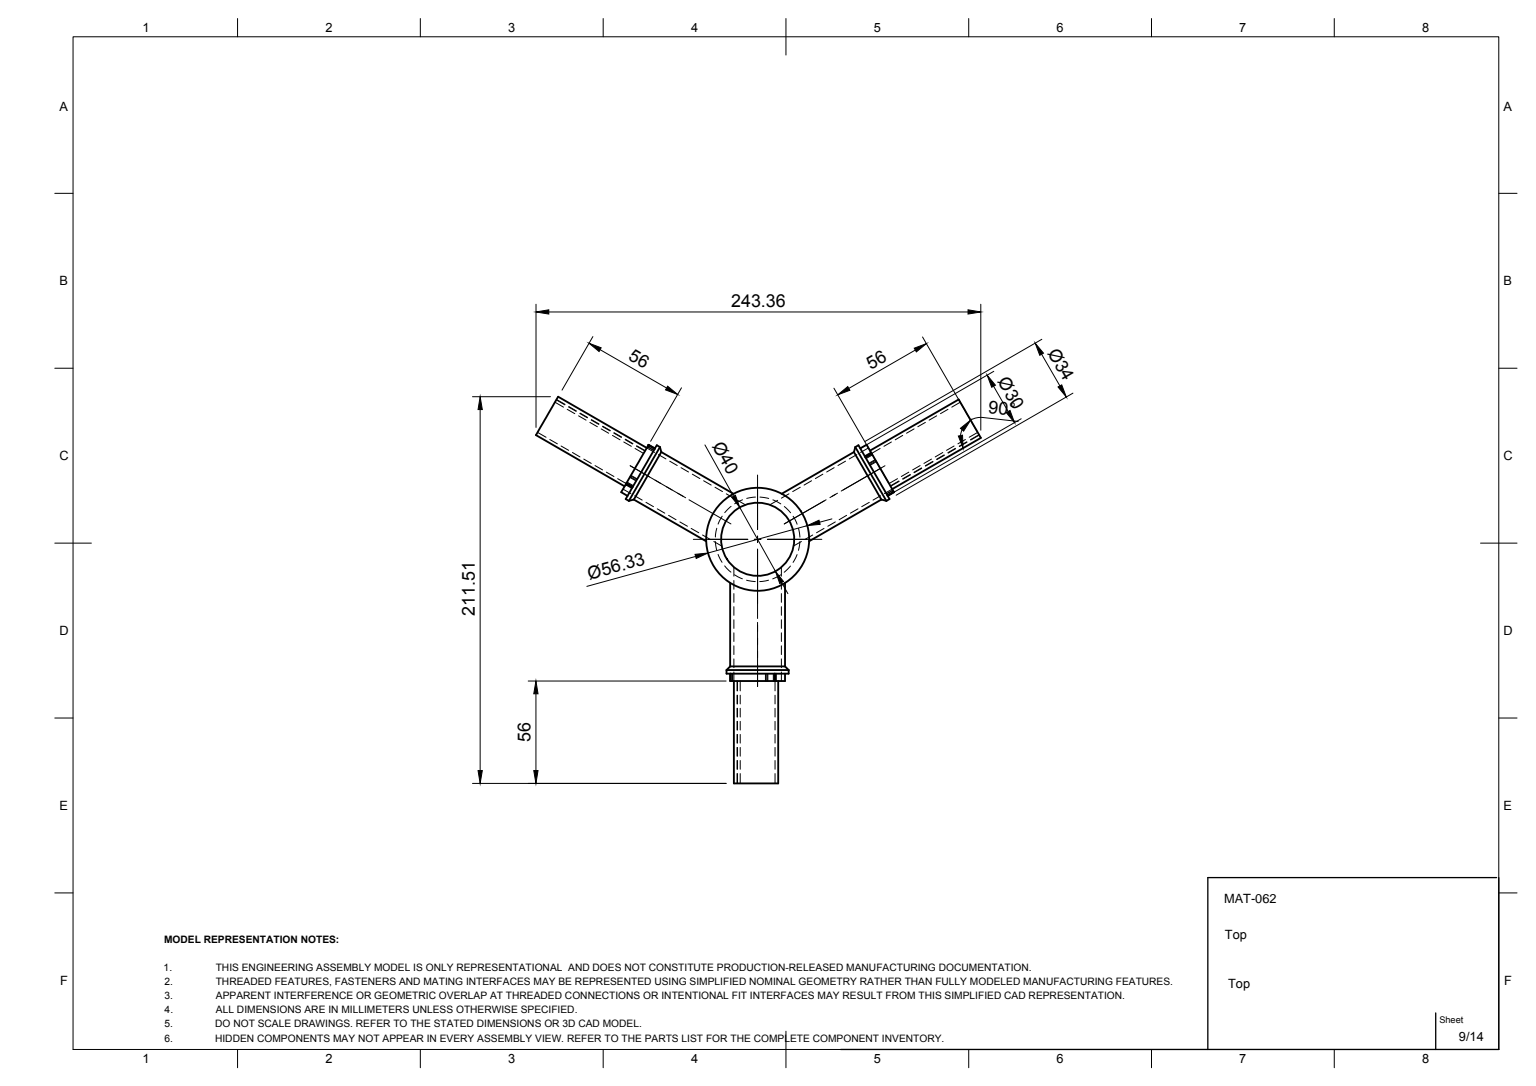
ISO-10303-21;
HEADER;
/* Generated by software containing ST-Developer
 * from STEP Tools, Inc. (www.steptools.com) 
 */

FILE_DESCRIPTION(
/* description */ (''),
/* implementation_level */ '2;1');

FILE_NAME(
/* name */ 'Top.step',
/* time_stamp */ '2026-10-24T10:18:25-07:00',
/* author */ (''),
/* organization */ (''),
/* preprocessor_version */ 'ST-DEVELOPER v20.2',
/* originating_system */ 'Autodesk Translation Framework v15.15.0.0',
/* authorisation */ '');

FILE_SCHEMA (('AUTOMOTIVE_DESIGN { 1 0 10303 214 3 1 1 }'));
ENDSEC;

DATA;
#10=MECHANICAL_DESIGN_GEOMETRIC_PRESENTATION_REPRESENTATION('',(#250,#251,#252,#253,#254,#255,#256,#257,#258,#259),#14125);
#191=CONICAL_SURFACE('',#6560,17.,0.785398163397448);
#192=CONICAL_SURFACE('',#6577,17.,0.785398163397452);
#193=CONICAL_SURFACE('',#6578,17.,0.785398163397448);
#230=SHAPE_REPRESENTATION_RELATIONSHIP('SRR','None',#14204,#240);
#240=ADVANCED_BREP_SHAPE_REPRESENTATION('',(#269,#270,#271,#272),#14118);
#250=STYLED_ITEM('',(#14263),#269);
#251=STYLED_ITEM('',(#14263),#270);
#252=STYLED_ITEM('',(#14263),#271);
#253=STYLED_ITEM('',(#14264),#5964);
#254=STYLED_ITEM('',(#14264),#5965);
#255=STYLED_ITEM('',(#14264),#5966);
#256=STYLED_ITEM('',(#14264),#5967);
#257=STYLED_ITEM('',(#14264),#5968);
#258=STYLED_ITEM('',(#14264),#5969);
#259=STYLED_ITEM('',(#14263),#272);
#269=MANIFOLD_SOLID_BREP('Top (1)',#6137);
#270=MANIFOLD_SOLID_BREP('Top (2)',#6138);
#271=MANIFOLD_SOLID_BREP('Top (3)',#6139);
#272=MANIFOLD_SOLID_BREP('Top (4)',#6140);
#395=B_SPLINE_CURVE_WITH_KNOTS('',3,(#11718,#11719,#11720,#11721,#11722,
#11723,#11724,#11725,#11726,#11727,#11728,#11729,#11730,#11731),
 .UNSPECIFIED.,.F.,.F.,(4,2,2,2,2,2,4),(9.25473526333439,9.54447442505159,
9.8342135867688,10.4136919102032,10.9910554946856,11.2797372869268,11.568419079168),
 .UNSPECIFIED.);
#396=B_SPLINE_CURVE_WITH_KNOTS('',3,(#11733,#11734,#11735,#11736,#11737,
#11738,#11739,#11740,#11741,#11742,#11743,#11744,#11745,#11746),
 .UNSPECIFIED.,.F.,.F.,(4,2,2,2,2,2,4),(6.94105144750079,7.22973323974199,
7.51841503198319,8.09577861646558,8.67525693989999,8.96499610161719,9.25473526333439),
 .UNSPECIFIED.);
#397=B_SPLINE_CURVE_WITH_KNOTS('',3,(#11751,#11752,#11753,#11754,#11755,
#11756,#11757,#11758,#11759,#11760,#11761,#11762,#11763,#11764),
 .UNSPECIFIED.,.F.,.F.,(4,2,2,2,2,2,4),(4.6273676316672,4.9171067933844,
5.2068459551016,5.78632427853601,6.3636878630184,6.6523696552596,6.94105144750079),
 .UNSPECIFIED.);
#398=B_SPLINE_CURVE_WITH_KNOTS('',3,(#11765,#11766,#11767,#11768,#11769,
#11770,#11771,#11772,#11773,#11774,#11775,#11776,#11777,#11778),
 .UNSPECIFIED.,.F.,.F.,(4,2,2,2,2,2,4),(11.568419079168,11.8571008714092,
12.1457826636504,12.7231462481328,13.3026245715672,13.5923637332844,13.8821028950016),
 .UNSPECIFIED.);
#399=B_SPLINE_CURVE_WITH_KNOTS('',3,(#11781,#11782,#11783,#11784,#11785,
#11786,#11787,#11788,#11789,#11790,#11791,#11792,#11793,#11794,#11795,#11796,
#11797,#11798,#11799,#11800,#11801,#11802,#11803,#11804,#11805,#11806),
 .UNSPECIFIED.,.F.,.F.,(4,2,2,2,2,2,2,2,2,2,2,2,4),(4.6273676316672,4.9171067933844,
5.2068459551016,5.78632427853601,6.3636878630184,6.6523696552596,6.94105144750079,
7.22973323974199,7.51841503198319,8.09577861646558,8.67525693989999,8.96499610161719,
9.25473526333439),.UNSPECIFIED.);
#400=B_SPLINE_CURVE_WITH_KNOTS('',3,(#11807,#11808,#11809,#11810,#11811,
#11812,#11813,#11814,#11815,#11816,#11817,#11818,#11819,#11820,#11821,#11822,
#11823,#11824,#11825,#11826,#11827,#11828,#11829,#11830,#11831,#11832),
 .UNSPECIFIED.,.F.,.F.,(4,2,2,2,2,2,2,2,2,2,2,2,4),(9.25473526333439,9.54447442505159,
9.8342135867688,10.4136919102032,10.9910554946856,11.2797372869268,11.568419079168,
11.8571008714092,12.1457826636504,12.7231462481328,13.3026245715672,13.5923637332844,
13.8821028950016),.UNSPECIFIED.);
#401=B_SPLINE_CURVE_WITH_KNOTS('',3,(#11835,#11836,#11837,#11838,#11839,
#11840,#11841,#11842,#11843,#11844,#11845,#11846,#11847,#11848,#11849,#11850,
#11851,#11852,#11853,#11854,#11855,#11856,#11857,#11858,#11859,#11860),
 .UNSPECIFIED.,.F.,.F.,(4,2,2,2,2,2,2,2,2,2,2,2,4),(4.62736763166719,4.9171067933844,
5.2068459551016,5.78632427853601,6.3636878630184,6.6523696552596,6.94105144750079,
7.22973323974199,7.51841503198319,8.09577861646558,8.67525693989998,8.96499610161719,
9.25473526333439),.UNSPECIFIED.);
#402=B_SPLINE_CURVE_WITH_KNOTS('',3,(#11861,#11862,#11863,#11864,#11865,
#11866,#11867,#11868,#11869,#11870,#11871,#11872,#11873,#11874,#11875,#11876,
#11877,#11878,#11879,#11880,#11881,#11882,#11883,#11884,#11885,#11886),
 .UNSPECIFIED.,.F.,.F.,(4,2,2,2,2,2,2,2,2,2,2,2,4),(9.25473526333439,9.54447442505159,
9.8342135867688,10.4136919102032,10.9910554946856,11.2797372869268,11.568419079168,
11.8571008714092,12.1457826636504,12.7231462481328,13.3026245715672,13.5923637332844,
13.8821028950016),.UNSPECIFIED.);
#403=B_SPLINE_CURVE_WITH_KNOTS('',3,(#11929,#11930,#11931,#11932,#11933,
#11934,#11935,#11936,#11937,#11938,#11939,#11940,#11941,#11942),
 .UNSPECIFIED.,.F.,.F.,(4,2,2,2,2,2,4),(-4.06985486860275,-3.8142561336285,
-3.55865739865425,-3.04745992870576,-2.54119368150357,-2.28806055790247,
-2.03492743430138),.UNSPECIFIED.);
#404=B_SPLINE_CURVE_WITH_KNOTS('',3,(#11944,#11945,#11946,#11947,#11948,
#11949,#11950,#11951,#11952,#11953,#11954,#11955,#11956,#11957),
 .UNSPECIFIED.,.F.,.F.,(4,2,2,2,2,2,4),(2.03492743430138,2.28806055790247,
2.54119368150357,3.04745992870576,3.55865739865425,3.8142561336285,4.06985486860275),
 .UNSPECIFIED.);
#405=B_SPLINE_CURVE_WITH_KNOTS('',3,(#11959,#11960,#11961,#11962,#11963,
#11964,#11965,#11966,#11967,#11968,#11969,#11970,#11971,#11972),
 .UNSPECIFIED.,.F.,.F.,(4,2,2,2,2,2,4),(0.,0.255598734974248,0.511197469948496,
1.02239493989699,1.52866118709918,1.78179431070028,2.03492743430138),
 .UNSPECIFIED.);
#406=B_SPLINE_CURVE_WITH_KNOTS('',3,(#11974,#11975,#11976,#11977,#11978,
#11979,#11980,#11981,#11982,#11983,#11984,#11985,#11986,#11987),
 .UNSPECIFIED.,.F.,.F.,(4,2,2,2,2,2,4),(-2.03492743430138,-1.78179431070028,
-1.52866118709918,-1.02239493989699,-0.511197469948497,-0.255598734974249,
0.),.UNSPECIFIED.);
#407=B_SPLINE_CURVE_WITH_KNOTS('',3,(#12049,#12050,#12051,#12052,#12053,
#12054,#12055,#12056,#12057,#12058,#12059,#12060,#12061,#12062,#12063,#12064,
#12065,#12066,#12067,#12068,#12069,#12070,#12071,#12072,#12073,#12074),
 .UNSPECIFIED.,.F.,.F.,(4,2,2,2,2,2,2,2,2,2,2,2,4),(-4.06985486860275,-3.8142561336285,
-3.55865739865425,-3.04745992870576,-2.54119368150357,-2.28806055790247,
-2.03492743430138,-1.78179431070028,-1.52866118709918,-1.02239493989699,
-0.511197469948497,-0.255598734974249,0.),.UNSPECIFIED.);
#408=B_SPLINE_CURVE_WITH_KNOTS('',3,(#12075,#12076,#12077,#12078,#12079,
#12080,#12081,#12082,#12083,#12084,#12085,#12086,#12087,#12088,#12089,#12090,
#12091,#12092,#12093,#12094,#12095,#12096,#12097,#12098,#12099,#12100),
 .UNSPECIFIED.,.F.,.F.,(4,2,2,2,2,2,2,2,2,2,2,2,4),(0.,0.255598734974248,
0.511197469948495,1.02239493989699,1.52866118709918,1.78179431070028,2.03492743430137,
2.28806055790247,2.54119368150357,3.04745992870576,3.55865739865425,3.8142561336285,
4.06985486860275),.UNSPECIFIED.);
#409=B_SPLINE_CURVE_WITH_KNOTS('',3,(#12105,#12106,#12107,#12108,#12109,
#12110,#12111,#12112,#12113,#12114,#12115,#12116,#12117,#12118,#12119,#12120,
#12121,#12122,#12123,#12124,#12125,#12126,#12127,#12128,#12129,#12130),
 .UNSPECIFIED.,.F.,.F.,(4,2,2,2,2,2,2,2,2,2,2,2,4),(-4.06985486860275,-3.8142561336285,
-3.55865739865425,-3.04745992870576,-2.54119368150357,-2.28806055790247,
-2.03492743430137,-1.78179431070028,-1.52866118709918,-1.02239493989699,
-0.511197469948497,-0.255598734974249,0.),.UNSPECIFIED.);
#410=B_SPLINE_CURVE_WITH_KNOTS('',3,(#12131,#12132,#12133,#12134,#12135,
#12136,#12137,#12138,#12139,#12140,#12141,#12142,#12143,#12144,#12145,#12146,
#12147,#12148,#12149,#12150,#12151,#12152,#12153,#12154,#12155,#12156),
 .UNSPECIFIED.,.F.,.F.,(4,2,2,2,2,2,2,2,2,2,2,2,4),(0.,0.255598734974248,
0.511197469948495,1.02239493989699,1.52866118709918,1.78179431070028,2.03492743430137,
2.28806055790247,2.54119368150357,3.04745992870576,3.55865739865425,3.8142561336285,
4.06985486860275),.UNSPECIFIED.);
#527=CYLINDRICAL_SURFACE('',#6483,10.9999999999984);
#528=CYLINDRICAL_SURFACE('',#6486,13.0000000000012);
#529=CYLINDRICAL_SURFACE('',#6493,10.9999999999984);
#530=CYLINDRICAL_SURFACE('',#6496,13.0000000000012);
#531=CYLINDRICAL_SURFACE('',#6503,10.9999999999984);
#532=CYLINDRICAL_SURFACE('',#6506,13.0000000000012);
#533=CYLINDRICAL_SURFACE('',#6509,15.);
#534=CYLINDRICAL_SURFACE('',#6512,15.);
#535=CYLINDRICAL_SURFACE('',#6515,15.);
#536=CYLINDRICAL_SURFACE('',#6520,15.);
#537=CYLINDRICAL_SURFACE('',#6523,15.);
#538=CYLINDRICAL_SURFACE('',#6526,15.);
#539=CYLINDRICAL_SURFACE('',#6531,15.);
#540=CYLINDRICAL_SURFACE('',#6534,15.);
#541=CYLINDRICAL_SURFACE('',#6537,15.);
#542=CYLINDRICAL_SURFACE('',#6542,28.1634258170599);
#543=CYLINDRICAL_SURFACE('',#6549,23.1634258170599);
#544=CYLINDRICAL_SURFACE('',#6552,15.);
#545=CYLINDRICAL_SURFACE('',#6556,17.);
#546=CYLINDRICAL_SURFACE('',#6559,13.);
#547=CYLINDRICAL_SURFACE('',#6561,15.);
#548=CYLINDRICAL_SURFACE('',#6563,15.);
#549=CYLINDRICAL_SURFACE('',#6567,17.);
#550=CYLINDRICAL_SURFACE('',#6572,17.);
#551=CYLINDRICAL_SURFACE('',#6575,13.);
#552=CYLINDRICAL_SURFACE('',#6576,13.);
#553=CYLINDRICAL_SURFACE('',#6581,20.);
#663=FACE_BOUND('',#1271,.T.);
#664=FACE_BOUND('',#1276,.T.);
#665=FACE_BOUND('',#1281,.T.);
#666=FACE_BOUND('',#1283,.T.);
#667=FACE_BOUND('',#1284,.T.);
#668=FACE_BOUND('',#1286,.T.);
#669=FACE_BOUND('',#1288,.T.);
#670=FACE_BOUND('',#1293,.T.);
#671=FACE_BOUND('',#1300,.T.);
#672=FACE_BOUND('',#1303,.T.);
#673=FACE_BOUND('',#1311,.T.);
#674=FACE_BOUND('',#1312,.T.);
#860=FACE_OUTER_BOUND('',#1249,.T.);
#861=FACE_OUTER_BOUND('',#1250,.T.);
#862=FACE_OUTER_BOUND('',#1251,.T.);
#863=FACE_OUTER_BOUND('',#1252,.T.);
#864=FACE_OUTER_BOUND('',#1253,.T.);
#865=FACE_OUTER_BOUND('',#1254,.T.);
#866=FACE_OUTER_BOUND('',#1255,.T.);
#867=FACE_OUTER_BOUND('',#1256,.T.);
#868=FACE_OUTER_BOUND('',#1257,.T.);
#869=FACE_OUTER_BOUND('',#1258,.T.);
#870=FACE_OUTER_BOUND('',#1259,.T.);
#871=FACE_OUTER_BOUND('',#1260,.T.);
#872=FACE_OUTER_BOUND('',#1261,.T.);
#873=FACE_OUTER_BOUND('',#1262,.T.);
#874=FACE_OUTER_BOUND('',#1263,.T.);
#875=FACE_OUTER_BOUND('',#1264,.T.);
#876=FACE_OUTER_BOUND('',#1265,.T.);
#877=FACE_OUTER_BOUND('',#1266,.T.);
#878=FACE_OUTER_BOUND('',#1267,.T.);
#879=FACE_OUTER_BOUND('',#1268,.T.);
#880=FACE_OUTER_BOUND('',#1269,.T.);
#881=FACE_OUTER_BOUND('',#1270,.T.);
#882=FACE_OUTER_BOUND('',#1272,.T.);
#883=FACE_OUTER_BOUND('',#1273,.T.);
#884=FACE_OUTER_BOUND('',#1274,.T.);
#885=FACE_OUTER_BOUND('',#1275,.T.);
#886=FACE_OUTER_BOUND('',#1277,.T.);
#887=FACE_OUTER_BOUND('',#1278,.T.);
#888=FACE_OUTER_BOUND('',#1279,.T.);
#889=FACE_OUTER_BOUND('',#1280,.T.);
#890=FACE_OUTER_BOUND('',#1282,.T.);
#891=FACE_OUTER_BOUND('',#1285,.T.);
#892=FACE_OUTER_BOUND('',#1287,.T.);
#893=FACE_OUTER_BOUND('',#1289,.T.);
#894=FACE_OUTER_BOUND('',#1290,.T.);
#895=FACE_OUTER_BOUND('',#1291,.T.);
#896=FACE_OUTER_BOUND('',#1292,.T.);
#897=FACE_OUTER_BOUND('',#1294,.T.);
#898=FACE_OUTER_BOUND('',#1295,.T.);
#899=FACE_OUTER_BOUND('',#1296,.T.);
#900=FACE_OUTER_BOUND('',#1297,.T.);
#901=FACE_OUTER_BOUND('',#1298,.T.);
#902=FACE_OUTER_BOUND('',#1299,.T.);
#903=FACE_OUTER_BOUND('',#1301,.T.);
#904=FACE_OUTER_BOUND('',#1302,.T.);
#905=FACE_OUTER_BOUND('',#1304,.T.);
#906=FACE_OUTER_BOUND('',#1305,.T.);
#907=FACE_OUTER_BOUND('',#1306,.T.);
#908=FACE_OUTER_BOUND('',#1307,.T.);
#909=FACE_OUTER_BOUND('',#1308,.T.);
#910=FACE_OUTER_BOUND('',#1309,.T.);
#911=FACE_OUTER_BOUND('',#1310,.T.);
#912=FACE_OUTER_BOUND('',#1313,.T.);
#913=FACE_OUTER_BOUND('',#1314,.T.);
#914=FACE_OUTER_BOUND('',#1315,.T.);
#915=FACE_OUTER_BOUND('',#1316,.T.);
#916=FACE_OUTER_BOUND('',#1317,.T.);
#917=FACE_OUTER_BOUND('',#1318,.T.);
#918=FACE_OUTER_BOUND('',#1319,.T.);
#919=FACE_OUTER_BOUND('',#1320,.T.);
#920=FACE_OUTER_BOUND('',#1321,.T.);
#921=FACE_OUTER_BOUND('',#1322,.T.);
#922=FACE_OUTER_BOUND('',#1323,.T.);
#923=FACE_OUTER_BOUND('',#1324,.T.);
#924=FACE_OUTER_BOUND('',#1325,.T.);
#925=FACE_OUTER_BOUND('',#1326,.T.);
#926=FACE_OUTER_BOUND('',#1327,.T.);
#927=FACE_OUTER_BOUND('',#1328,.T.);
#928=FACE_OUTER_BOUND('',#1329,.T.);
#929=FACE_OUTER_BOUND('',#1330,.T.);
#930=FACE_OUTER_BOUND('',#1331,.T.);
#931=FACE_OUTER_BOUND('',#1332,.T.);
#932=FACE_OUTER_BOUND('',#1333,.T.);
#933=FACE_OUTER_BOUND('',#1334,.T.);
#934=FACE_OUTER_BOUND('',#1335,.T.);
#935=FACE_OUTER_BOUND('',#1336,.T.);
#936=FACE_OUTER_BOUND('',#1337,.T.);
#937=FACE_OUTER_BOUND('',#1338,.T.);
#938=FACE_OUTER_BOUND('',#1339,.T.);
#1249=EDGE_LOOP('',(#4585,#4586,#4587,#4588));
#1250=EDGE_LOOP('',(#4589,#4590,#4591,#4592));
#1251=EDGE_LOOP('',(#4593,#4594,#4595,#4596));
#1252=EDGE_LOOP('',(#4597,#4598,#4599,#4600));
#1253=EDGE_LOOP('',(#4601,#4602,#4603,#4604));
#1254=EDGE_LOOP('',(#4605,#4606,#4607,#4608));
#1255=EDGE_LOOP('',(#4609,#4610,#4611,#4612));
#1256=EDGE_LOOP('',(#4613,#4614,#4615,#4616));
#1257=EDGE_LOOP('',(#4617,#4618,#4619,#4620));
#1258=EDGE_LOOP('',(#4621,#4622,#4623,#4624));
#1259=EDGE_LOOP('',(#4625,#4626,#4627,#4628));
#1260=EDGE_LOOP('',(#4629,#4630,#4631,#4632));
#1261=EDGE_LOOP('',(#4633,#4634,#4635,#4636));
#1262=EDGE_LOOP('',(#4637,#4638,#4639,#4640));
#1263=EDGE_LOOP('',(#4641,#4642,#4643,#4644));
#1264=EDGE_LOOP('',(#4645,#4646,#4647,#4648));
#1265=EDGE_LOOP('',(#4649,#4650,#4651,#4652));
#1266=EDGE_LOOP('',(#4653,#4654,#4655,#4656));
#1267=EDGE_LOOP('',(#4657,#4658,#4659,#4660));
#1268=EDGE_LOOP('',(#4661,#4662,#4663,#4664));
#1269=EDGE_LOOP('',(#4665,#4666,#4667,#4668));
#1270=EDGE_LOOP('',(#4669,#4670,#4671,#4672,#4673,#4674,#4675,#4676,#4677,
#4678,#4679,#4680));
#1271=EDGE_LOOP('',(#4681));
#1272=EDGE_LOOP('',(#4682,#4683,#4684,#4685));
#1273=EDGE_LOOP('',(#4686,#4687,#4688,#4689));
#1274=EDGE_LOOP('',(#4690,#4691,#4692,#4693));
#1275=EDGE_LOOP('',(#4694,#4695,#4696,#4697,#4698,#4699,#4700,#4701,#4702,
#4703,#4704,#4705));
#1276=EDGE_LOOP('',(#4706));
#1277=EDGE_LOOP('',(#4707,#4708,#4709,#4710));
#1278=EDGE_LOOP('',(#4711,#4712,#4713,#4714));
#1279=EDGE_LOOP('',(#4715,#4716,#4717,#4718));
#1280=EDGE_LOOP('',(#4719,#4720,#4721,#4722,#4723,#4724,#4725,#4726,#4727,
#4728,#4729,#4730));
#1281=EDGE_LOOP('',(#4731));
#1282=EDGE_LOOP('',(#4732,#4733,#4734,#4735,#4736,#4737,#4738,#4739,#4740,
#4741));
#1283=EDGE_LOOP('',(#4742,#4743));
#1284=EDGE_LOOP('',(#4744,#4745));
#1285=EDGE_LOOP('',(#4746));
#1286=EDGE_LOOP('',(#4747));
#1287=EDGE_LOOP('',(#4748));
#1288=EDGE_LOOP('',(#4749));
#1289=EDGE_LOOP('',(#4750,#4751,#4752,#4753));
#1290=EDGE_LOOP('',(#4754));
#1291=EDGE_LOOP('',(#4755,#4756,#4757,#4758,#4759,#4760,#4761));
#1292=EDGE_LOOP('',(#4762));
#1293=EDGE_LOOP('',(#4763,#4764,#4765,#4766,#4767,#4768,#4769,#4770,#4771,
#4772,#4773,#4774));
#1294=EDGE_LOOP('',(#4775,#4776,#4777,#4778,#4779));
#1295=EDGE_LOOP('',(#4780,#4781,#4782,#4783,#4784,#4785,#4786));
#1296=EDGE_LOOP('',(#4787,#4788,#4789,#4790,#4791));
#1297=EDGE_LOOP('',(#4792,#4793,#4794,#4795,#4796));
#1298=EDGE_LOOP('',(#4797,#4798,#4799,#4800,#4801));
#1299=EDGE_LOOP('',(#4802));
#1300=EDGE_LOOP('',(#4803,#4804,#4805,#4806,#4807,#4808,#4809,#4810,#4811,
#4812,#4813,#4814));
#1301=EDGE_LOOP('',(#4815,#4816,#4817,#4818,#4819));
#1302=EDGE_LOOP('',(#4820));
#1303=EDGE_LOOP('',(#4821,#4822,#4823,#4824,#4825,#4826,#4827,#4828,#4829,
#4830,#4831,#4832));
#1304=EDGE_LOOP('',(#4833,#4834,#4835,#4836,#4837));
#1305=EDGE_LOOP('',(#4838,#4839,#4840,#4841,#4842));
#1306=EDGE_LOOP('',(#4843,#4844,#4845,#4846,#4847));
#1307=EDGE_LOOP('',(#4848,#4849,#4850,#4851,#4852));
#1308=EDGE_LOOP('',(#4853,#4854,#4855,#4856,#4857));
#1309=EDGE_LOOP('',(#4858));
#1310=EDGE_LOOP('',(#4859,#4860,#4861,#4862,#4863,#4864,#4865,#4866,#4867,
#4868));
#1311=EDGE_LOOP('',(#4869,#4870));
#1312=EDGE_LOOP('',(#4871,#4872));
#1313=EDGE_LOOP('',(#4873,#4874,#4875,#4876));
#1314=EDGE_LOOP('',(#4877,#4878,#4879,#4880));
#1315=EDGE_LOOP('',(#4881,#4882,#4883,#4884));
#1316=EDGE_LOOP('',(#4885,#4886,#4887,#4888));
#1317=EDGE_LOOP('',(#4889,#4890,#4891,#4892));
#1318=EDGE_LOOP('',(#4893,#4894,#4895,#4896));
#1319=EDGE_LOOP('',(#4897,#4898,#4899,#4900));
#1320=EDGE_LOOP('',(#4901,#4902,#4903,#4904));
#1321=EDGE_LOOP('',(#4905,#4906,#4907,#4908));
#1322=EDGE_LOOP('',(#4909,#4910,#4911,#4912));
#1323=EDGE_LOOP('',(#4913,#4914,#4915,#4916));
#1324=EDGE_LOOP('',(#4917,#4918,#4919,#4920));
#1325=EDGE_LOOP('',(#4921,#4922,#4923,#4924));
#1326=EDGE_LOOP('',(#4925,#4926,#4927,#4928));
#1327=EDGE_LOOP('',(#4929,#4930,#4931,#4932));
#1328=EDGE_LOOP('',(#4933,#4934,#4935,#4936));
#1329=EDGE_LOOP('',(#4937,#4938,#4939,#4940));
#1330=EDGE_LOOP('',(#4941,#4942,#4943,#4944));
#1331=EDGE_LOOP('',(#4945,#4946,#4947,#4948));
#1332=EDGE_LOOP('',(#4949,#4950,#4951,#4952));
#1333=EDGE_LOOP('',(#4953,#4954,#4955,#4956));
#1334=EDGE_LOOP('',(#4957,#4958,#4959,#4960));
#1335=EDGE_LOOP('',(#4961,#4962,#4963,#4964));
#1336=EDGE_LOOP('',(#4965,#4966,#4967,#4968));
#1337=EDGE_LOOP('',(#4969,#4970,#4971,#4972));
#1338=EDGE_LOOP('',(#4973,#4974,#4975,#4976));
#1339=EDGE_LOOP('',(#4977,#4978,#4979,#4980));
#1648=CIRCLE('',#6480,13.0000000000012);
#1649=CIRCLE('',#6481,10.9999999999984);
#1650=CIRCLE('',#6484,10.9999999999984);
#1651=CIRCLE('',#6487,13.);
#1652=CIRCLE('',#6490,13.0000000000012);
#1653=CIRCLE('',#6491,10.9999999999984);
#1654=CIRCLE('',#6494,10.9999999999984);
#1655=CIRCLE('',#6497,13.);
#1656=CIRCLE('',#6500,13.0000000000012);
#1657=CIRCLE('',#6501,10.9999999999984);
#1658=CIRCLE('',#6504,10.9999999999984);
#1659=CIRCLE('',#6507,13.);
#1660=CIRCLE('',#6510,15.);
#1661=CIRCLE('',#6511,15.);
#1662=CIRCLE('',#6513,15.);
#1663=CIRCLE('',#6514,15.);
#1664=CIRCLE('',#6516,15.);
#1665=CIRCLE('',#6517,15.);
#1666=CIRCLE('',#6519,13.);
#1667=CIRCLE('',#6521,15.);
#1668=CIRCLE('',#6522,15.);
#1669=CIRCLE('',#6524,15.);
#1670=CIRCLE('',#6525,15.);
#1671=CIRCLE('',#6527,15.);
#1672=CIRCLE('',#6528,15.);
#1673=CIRCLE('',#6530,13.);
#1674=CIRCLE('',#6532,15.);
#1675=CIRCLE('',#6533,15.);
#1676=CIRCLE('',#6535,15.);
#1677=CIRCLE('',#6536,15.);
#1678=CIRCLE('',#6538,15.);
#1679=CIRCLE('',#6539,15.);
#1680=CIRCLE('',#6541,13.);
#1681=CIRCLE('',#6543,28.1634258170599);
#1682=CIRCLE('',#6544,28.1634258170599);
#1683=CIRCLE('',#6546,23.1634258170599);
#1684=CIRCLE('',#6548,20.);
#1685=CIRCLE('',#6550,23.1634258170599);
#1686=CIRCLE('',#6553,15.);
#1687=CIRCLE('',#6555,17.);
#1688=CIRCLE('',#6557,17.);
#1689=CIRCLE('',#6558,17.);
#1690=CIRCLE('',#6562,15.);
#1691=CIRCLE('',#6564,15.);
#1692=CIRCLE('',#6566,17.);
#1693=CIRCLE('',#6568,17.);
#1694=CIRCLE('',#6569,17.);
#1695=CIRCLE('',#6571,17.);
#1696=CIRCLE('',#6573,17.);
#1697=CIRCLE('',#6574,17.);
#1698=CIRCLE('',#6580,20.);
#1907=LINE('',#11504,#2295);
#1908=LINE('',#11507,#2296);
#1909=LINE('',#11511,#2297);
#1910=LINE('',#11512,#2298);
#1911=LINE('',#11513,#2299);
#1912=LINE('',#11517,#2300);
#1913=LINE('',#11520,#2301);
#1914=LINE('',#11521,#2302);
#1915=LINE('',#11530,#2303);
#1916=LINE('',#11533,#2304);
#1917=LINE('',#11537,#2305);
#1918=LINE('',#11538,#2306);
#1919=LINE('',#11539,#2307);
#1920=LINE('',#11543,#2308);
#1921=LINE('',#11546,#2309);
#1922=LINE('',#11547,#2310);
#1923=LINE('',#11556,#2311);
#1924=LINE('',#11559,#2312);
#1925=LINE('',#11563,#2313);
#1926=LINE('',#11564,#2314);
#1927=LINE('',#11565,#2315);
#1928=LINE('',#11569,#2316);
#1929=LINE('',#11572,#2317);
#1930=LINE('',#11573,#2318);
#1931=LINE('',#11580,#2319);
#1932=LINE('',#11584,#2320);
#1933=LINE('',#11589,#2321);
#1934=LINE('',#11593,#2322);
#1935=LINE('',#11598,#2323);
#1936=LINE('',#11602,#2324);
#1937=LINE('',#11606,#2325);
#1938=LINE('',#11608,#2326);
#1939=LINE('',#11609,#2327);
#1940=LINE('',#11611,#2328);
#1941=LINE('',#11613,#2329);
#1942=LINE('',#11614,#2330);
#1943=LINE('',#11616,#2331);
#1944=LINE('',#11618,#2332);
#1945=LINE('',#11619,#2333);
#1946=LINE('',#11625,#2334);
#1947=LINE('',#11629,#2335);
#1948=LINE('',#11634,#2336);
#1949=LINE('',#11638,#2337);
#1950=LINE('',#11643,#2338);
#1951=LINE('',#11647,#2339);
#1952=LINE('',#11651,#2340);
#1953=LINE('',#11653,#2341);
#1954=LINE('',#11654,#2342);
#1955=LINE('',#11656,#2343);
#1956=LINE('',#11658,#2344);
#1957=LINE('',#11659,#2345);
#1958=LINE('',#11661,#2346);
#1959=LINE('',#11663,#2347);
#1960=LINE('',#11664,#2348);
#1961=LINE('',#11670,#2349);
#1962=LINE('',#11674,#2350);
#1963=LINE('',#11679,#2351);
#1964=LINE('',#11683,#2352);
#1965=LINE('',#11688,#2353);
#1966=LINE('',#11692,#2354);
#1967=LINE('',#11696,#2355);
#1968=LINE('',#11698,#2356);
#1969=LINE('',#11699,#2357);
#1970=LINE('',#11701,#2358);
#1971=LINE('',#11703,#2359);
#1972=LINE('',#11704,#2360);
#1973=LINE('',#11706,#2361);
#1974=LINE('',#11708,#2362);
#1975=LINE('',#11709,#2363);
#1976=LINE('',#11716,#2364);
#1977=LINE('',#11748,#2365);
#1978=LINE('',#11896,#2366);
#1979=LINE('',#11901,#2367);
#1980=LINE('',#11906,#2368);
#1981=LINE('',#11908,#2369);
#1982=LINE('',#11909,#2370);
#1983=LINE('',#11911,#2371);
#1984=LINE('',#11913,#2372);
#1985=LINE('',#11914,#2373);
#1986=LINE('',#11916,#2374);
#1987=LINE('',#11918,#2375);
#1988=LINE('',#11919,#2376);
#1989=LINE('',#11925,#2377);
#1990=LINE('',#11973,#2378);
#1991=LINE('',#11989,#2379);
#1992=LINE('',#11993,#2380);
#1993=LINE('',#11997,#2381);
#1994=LINE('',#12002,#2382);
#1995=LINE('',#12004,#2383);
#1996=LINE('',#12006,#2384);
#1997=LINE('',#12007,#2385);
#1998=LINE('',#12009,#2386);
#1999=LINE('',#12011,#2387);
#2000=LINE('',#12012,#2388);
#2001=LINE('',#12014,#2389);
#2002=LINE('',#12015,#2390);
#2003=LINE('',#12021,#2391);
#2004=LINE('',#12026,#2392);
#2005=LINE('',#12028,#2393);
#2006=LINE('',#12030,#2394);
#2007=LINE('',#12031,#2395);
#2008=LINE('',#12033,#2396);
#2009=LINE('',#12035,#2397);
#2010=LINE('',#12036,#2398);
#2011=LINE('',#12038,#2399);
#2012=LINE('',#12039,#2400);
#2013=LINE('',#12045,#2401);
#2014=LINE('',#12101,#2402);
#2015=LINE('',#12157,#2403);
#2016=LINE('',#12159,#2404);
#2017=LINE('',#12161,#2405);
#2018=LINE('',#12166,#2406);
#2019=LINE('',#12167,#2407);
#2020=LINE('',#12169,#2408);
#2021=LINE('',#12171,#2409);
#2022=LINE('',#12174,#2410);
#2023=LINE('',#12176,#2411);
#2024=LINE('',#12179,#2412);
#2025=LINE('',#12181,#2413);
#2026=LINE('',#12184,#2414);
#2027=LINE('',#12186,#2415);
#2028=LINE('',#12189,#2416);
#2029=LINE('',#12191,#2417);
#2030=LINE('',#12194,#2418);
#2031=LINE('',#12196,#2419);
#2032=LINE('',#12199,#2420);
#2033=LINE('',#12201,#2421);
#2034=LINE('',#12204,#2422);
#2035=LINE('',#12206,#2423);
#2036=LINE('',#12209,#2424);
#2037=LINE('',#12211,#2425);
#2295=VECTOR('',#7457,2.00000000000281);
#2296=VECTOR('',#7460,2.00000000000281);
#2297=VECTOR('',#7463,1.99999999999748);
#2298=VECTOR('',#7464,55.9999999999999);
#2299=VECTOR('',#7465,55.9999999999999);
#2300=VECTOR('',#7470,56.0000000000002);
#2301=VECTOR('',#7473,2.0000000000017);
#2302=VECTOR('',#7474,56.0000000000002);
#2303=VECTOR('',#7485,2.0000000000028);
#2304=VECTOR('',#7488,2.00000000000279);
#2305=VECTOR('',#7491,2.00000000000043);
#2306=VECTOR('',#7492,56.);
#2307=VECTOR('',#7493,56.);
#2308=VECTOR('',#7498,56.);
#2309=VECTOR('',#7501,2.0000000000028);
#2310=VECTOR('',#7502,56.);
#2311=VECTOR('',#7513,2.0000000000028);
#2312=VECTOR('',#7516,2.00000000000278);
#2313=VECTOR('',#7519,1.99999999999811);
#2314=VECTOR('',#7520,55.9999999999998);
#2315=VECTOR('',#7521,55.9999999999998);
#2316=VECTOR('',#7526,56.0000000000001);
#2317=VECTOR('',#7529,2.00000000000235);
#2318=VECTOR('',#7530,56.0000000000001);
#2319=VECTOR('',#7539,4.);
#2320=VECTOR('',#7542,4.);
#2321=VECTOR('',#7547,4.);
#2322=VECTOR('',#7550,3.99999999999998);
#2323=VECTOR('',#7555,4.);
#2324=VECTOR('',#7558,3.99999999999998);
#2325=VECTOR('',#7563,1.04078523274219);
#2326=VECTOR('',#7564,1.0000000000001);
#2327=VECTOR('',#7565,1.04078523274216);
#2328=VECTOR('',#7566,1.04078523274217);
#2329=VECTOR('',#7567,0.999999999999985);
#2330=VECTOR('',#7568,1.04078523274216);
#2331=VECTOR('',#7569,1.04078523274218);
#2332=VECTOR('',#7570,1.);
#2333=VECTOR('',#7571,1.04078523274217);
#2334=VECTOR('',#7576,4.00000000000002);
#2335=VECTOR('',#7579,3.99999999999999);
#2336=VECTOR('',#7584,4.);
#2337=VECTOR('',#7587,4.00000000000005);
#2338=VECTOR('',#7592,4.00000000000001);
#2339=VECTOR('',#7595,4.);
#2340=VECTOR('',#7600,1.04078523274219);
#2341=VECTOR('',#7601,1.0000000000001);
#2342=VECTOR('',#7602,1.04078523274216);
#2343=VECTOR('',#7603,1.04078523274223);
#2344=VECTOR('',#7604,0.99999999999995);
#2345=VECTOR('',#7605,1.04078523274216);
#2346=VECTOR('',#7606,1.04078523274216);
#2347=VECTOR('',#7607,1.00000000000002);
#2348=VECTOR('',#7608,1.04078523274214);
#2349=VECTOR('',#7613,4.);
#2350=VECTOR('',#7616,4.);
#2351=VECTOR('',#7621,4.);
#2352=VECTOR('',#7624,4.);
#2353=VECTOR('',#7629,4.);
#2354=VECTOR('',#7632,4.);
#2355=VECTOR('',#7637,1.0407852327422);
#2356=VECTOR('',#7638,1.00000000000002);
#2357=VECTOR('',#7639,1.04078523274213);
#2358=VECTOR('',#7640,1.04078523274222);
#2359=VECTOR('',#7641,1.00000000000002);
#2360=VECTOR('',#7642,1.04078523274215);
#2361=VECTOR('',#7643,1.0407852327422);
#2362=VECTOR('',#7644,0.999999999999994);
#2363=VECTOR('',#7645,1.04078523274217);
#2364=VECTOR('',#7652,28.1634258170599);
#2365=VECTOR('',#7653,28.1634258170599);
#2366=VECTOR('',#7668,23.1634258170599);
#2367=VECTOR('',#7675,15.);
#2368=VECTOR('',#7680,1.04078523274216);
#2369=VECTOR('',#7681,1.);
#2370=VECTOR('',#7682,1.0407852327422);
#2371=VECTOR('',#7683,1.0407852327422);
#2372=VECTOR('',#7684,1.);
#2373=VECTOR('',#7685,1.0407852327422);
#2374=VECTOR('',#7686,1.04078523274218);
#2375=VECTOR('',#7687,1.);
#2376=VECTOR('',#7688,1.04078523274223);
#2377=VECTOR('',#7695,17.);
#2378=VECTOR('',#7698,13.);
#2379=VECTOR('',#7701,17.);
#2380=VECTOR('',#7706,15.);
#2381=VECTOR('',#7711,15.);
#2382=VECTOR('',#7716,1.0407852327422);
#2383=VECTOR('',#7717,1.04078523274217);
#2384=VECTOR('',#7718,1.);
#2385=VECTOR('',#7719,1.0407852327422);
#2386=VECTOR('',#7720,1.04078523274218);
#2387=VECTOR('',#7721,1.);
#2388=VECTOR('',#7722,1.0407852327422);
#2389=VECTOR('',#7723,1.0407852327422);
#2390=VECTOR('',#7724,1.00000000000001);
#2391=VECTOR('',#7731,17.);
#2392=VECTOR('',#7736,1.0407852327422);
#2393=VECTOR('',#7737,1.04078523274218);
#2394=VECTOR('',#7738,1.00000000000002);
#2395=VECTOR('',#7739,1.04078523274219);
#2396=VECTOR('',#7740,1.0407852327422);
#2397=VECTOR('',#7741,1.);
#2398=VECTOR('',#7742,1.04078523274225);
#2399=VECTOR('',#7743,1.0407852327422);
#2400=VECTOR('',#7744,1.00000000000001);
#2401=VECTOR('',#7751,17.);
#2402=VECTOR('',#7754,13.);
#2403=VECTOR('',#7757,13.);
#2404=VECTOR('',#7760,17.);
#2405=VECTOR('',#7763,17.);
#2406=VECTOR('',#7770,20.);
#2407=VECTOR('',#7771,20.);
#2408=VECTOR('',#7774,4.);
#2409=VECTOR('',#7777,4.);
#2410=VECTOR('',#7782,4.);
#2411=VECTOR('',#7785,4.);
#2412=VECTOR('',#7790,4.);
#2413=VECTOR('',#7793,4.);
#2414=VECTOR('',#7798,4.);
#2415=VECTOR('',#7801,4.);
#2416=VECTOR('',#7806,4.00000000000005);
#2417=VECTOR('',#7809,4.00000000000003);
#2418=VECTOR('',#7814,4.00000000000002);
#2419=VECTOR('',#7817,4.);
#2420=VECTOR('',#7822,4.);
#2421=VECTOR('',#7825,4.);
#2422=VECTOR('',#7830,4.);
#2423=VECTOR('',#7833,4.);
#2424=VECTOR('',#7838,3.99999999999998);
#2425=VECTOR('',#7841,3.99999999999998);
#2783=VERTEX_POINT('',#11500);
#2784=VERTEX_POINT('',#11501);
#2785=VERTEX_POINT('',#11503);
#2786=VERTEX_POINT('',#11505);
#2787=VERTEX_POINT('',#11509);
#2788=VERTEX_POINT('',#11510);
#2789=VERTEX_POINT('',#11515);
#2790=VERTEX_POINT('',#11519);
#2791=VERTEX_POINT('',#11526);
#2792=VERTEX_POINT('',#11527);
#2793=VERTEX_POINT('',#11529);
#2794=VERTEX_POINT('',#11531);
#2795=VERTEX_POINT('',#11535);
#2796=VERTEX_POINT('',#11536);
#2797=VERTEX_POINT('',#11541);
#2798=VERTEX_POINT('',#11545);
#2799=VERTEX_POINT('',#11552);
#2800=VERTEX_POINT('',#11553);
#2801=VERTEX_POINT('',#11555);
#2802=VERTEX_POINT('',#11557);
#2803=VERTEX_POINT('',#11561);
#2804=VERTEX_POINT('',#11562);
#2805=VERTEX_POINT('',#11567);
#2806=VERTEX_POINT('',#11571);
#2807=VERTEX_POINT('',#11578);
#2808=VERTEX_POINT('',#11579);
#2809=VERTEX_POINT('',#11581);
#2810=VERTEX_POINT('',#11583);
#2811=VERTEX_POINT('',#11587);
#2812=VERTEX_POINT('',#11588);
#2813=VERTEX_POINT('',#11590);
#2814=VERTEX_POINT('',#11592);
#2815=VERTEX_POINT('',#11596);
#2816=VERTEX_POINT('',#11597);
#2817=VERTEX_POINT('',#11599);
#2818=VERTEX_POINT('',#11601);
#2819=VERTEX_POINT('',#11605);
#2820=VERTEX_POINT('',#11607);
#2821=VERTEX_POINT('',#11610);
#2822=VERTEX_POINT('',#11612);
#2823=VERTEX_POINT('',#11615);
#2824=VERTEX_POINT('',#11617);
#2825=VERTEX_POINT('',#11620);
#2826=VERTEX_POINT('',#11623);
#2827=VERTEX_POINT('',#11624);
#2828=VERTEX_POINT('',#11626);
#2829=VERTEX_POINT('',#11628);
#2830=VERTEX_POINT('',#11632);
#2831=VERTEX_POINT('',#11633);
#2832=VERTEX_POINT('',#11635);
#2833=VERTEX_POINT('',#11637);
#2834=VERTEX_POINT('',#11641);
#2835=VERTEX_POINT('',#11642);
#2836=VERTEX_POINT('',#11644);
#2837=VERTEX_POINT('',#11646);
#2838=VERTEX_POINT('',#11650);
#2839=VERTEX_POINT('',#11652);
#2840=VERTEX_POINT('',#11655);
#2841=VERTEX_POINT('',#11657);
#2842=VERTEX_POINT('',#11660);
#2843=VERTEX_POINT('',#11662);
#2844=VERTEX_POINT('',#11665);
#2845=VERTEX_POINT('',#11668);
#2846=VERTEX_POINT('',#11669);
#2847=VERTEX_POINT('',#11671);
#2848=VERTEX_POINT('',#11673);
#2849=VERTEX_POINT('',#11677);
#2850=VERTEX_POINT('',#11678);
#2851=VERTEX_POINT('',#11680);
#2852=VERTEX_POINT('',#11682);
#2853=VERTEX_POINT('',#11686);
#2854=VERTEX_POINT('',#11687);
#2855=VERTEX_POINT('',#11689);
#2856=VERTEX_POINT('',#11691);
#2857=VERTEX_POINT('',#11695);
#2858=VERTEX_POINT('',#11697);
#2859=VERTEX_POINT('',#11700);
#2860=VERTEX_POINT('',#11702);
#2861=VERTEX_POINT('',#11705);
#2862=VERTEX_POINT('',#11707);
#2863=VERTEX_POINT('',#11710);
#2864=VERTEX_POINT('',#11713);
#2865=VERTEX_POINT('',#11715);
#2866=VERTEX_POINT('',#11717);
#2867=VERTEX_POINT('',#11732);
#2868=VERTEX_POINT('',#11747);
#2869=VERTEX_POINT('',#11750);
#2870=VERTEX_POINT('',#11779);
#2871=VERTEX_POINT('',#11780);
#2872=VERTEX_POINT('',#11833);
#2873=VERTEX_POINT('',#11834);
#2874=VERTEX_POINT('',#11888);
#2875=VERTEX_POINT('',#11891);
#2876=VERTEX_POINT('',#11894);
#2877=VERTEX_POINT('',#11899);
#2878=VERTEX_POINT('',#11903);
#2879=VERTEX_POINT('',#11905);
#2880=VERTEX_POINT('',#11907);
#2881=VERTEX_POINT('',#11910);
#2882=VERTEX_POINT('',#11912);
#2883=VERTEX_POINT('',#11915);
#2884=VERTEX_POINT('',#11917);
#2885=VERTEX_POINT('',#11921);
#2886=VERTEX_POINT('',#11922);
#2887=VERTEX_POINT('',#11927);
#2888=VERTEX_POINT('',#11928);
#2889=VERTEX_POINT('',#11943);
#2890=VERTEX_POINT('',#11958);
#2891=VERTEX_POINT('',#11991);
#2892=VERTEX_POINT('',#11995);
#2893=VERTEX_POINT('',#11999);
#2894=VERTEX_POINT('',#12001);
#2895=VERTEX_POINT('',#12003);
#2896=VERTEX_POINT('',#12005);
#2897=VERTEX_POINT('',#12008);
#2898=VERTEX_POINT('',#12010);
#2899=VERTEX_POINT('',#12013);
#2900=VERTEX_POINT('',#12017);
#2901=VERTEX_POINT('',#12018);
#2902=VERTEX_POINT('',#12023);
#2903=VERTEX_POINT('',#12025);
#2904=VERTEX_POINT('',#12027);
#2905=VERTEX_POINT('',#12029);
#2906=VERTEX_POINT('',#12032);
#2907=VERTEX_POINT('',#12034);
#2908=VERTEX_POINT('',#12037);
#2909=VERTEX_POINT('',#12041);
#2910=VERTEX_POINT('',#12042);
#2911=VERTEX_POINT('',#12047);
#2912=VERTEX_POINT('',#12048);
#2913=VERTEX_POINT('',#12103);
#2914=VERTEX_POINT('',#12104);
#2915=VERTEX_POINT('',#12163);
#3440=EDGE_CURVE('',#2783,#2784,#1648,.T.);
#3441=EDGE_CURVE('',#2784,#2785,#1907,.T.);
#3442=EDGE_CURVE('',#2785,#2786,#1649,.T.);
#3443=EDGE_CURVE('',#2786,#2783,#1908,.T.);
#3444=EDGE_CURVE('',#2787,#2788,#1909,.T.);
#3445=EDGE_CURVE('',#2787,#2785,#1910,.T.);
#3446=EDGE_CURVE('',#2788,#2784,#1911,.T.);
#3447=EDGE_CURVE('',#2789,#2787,#1650,.T.);
#3448=EDGE_CURVE('',#2789,#2786,#1912,.T.);
#3449=EDGE_CURVE('',#2790,#2789,#1913,.T.);
#3450=EDGE_CURVE('',#2790,#2783,#1914,.T.);
#3451=EDGE_CURVE('',#2788,#2790,#1651,.F.);
#3452=EDGE_CURVE('',#2791,#2792,#1652,.T.);
#3453=EDGE_CURVE('',#2792,#2793,#1915,.T.);
#3454=EDGE_CURVE('',#2793,#2794,#1653,.T.);
#3455=EDGE_CURVE('',#2794,#2791,#1916,.T.);
#3456=EDGE_CURVE('',#2795,#2796,#1917,.T.);
#3457=EDGE_CURVE('',#2795,#2793,#1918,.T.);
#3458=EDGE_CURVE('',#2796,#2792,#1919,.T.);
#3459=EDGE_CURVE('',#2797,#2795,#1654,.T.);
#3460=EDGE_CURVE('',#2797,#2794,#1920,.T.);
#3461=EDGE_CURVE('',#2798,#2797,#1921,.T.);
#3462=EDGE_CURVE('',#2798,#2791,#1922,.T.);
#3463=EDGE_CURVE('',#2796,#2798,#1655,.F.);
#3464=EDGE_CURVE('',#2799,#2800,#1656,.T.);
#3465=EDGE_CURVE('',#2800,#2801,#1923,.T.);
#3466=EDGE_CURVE('',#2801,#2802,#1657,.T.);
#3467=EDGE_CURVE('',#2802,#2799,#1924,.T.);
#3468=EDGE_CURVE('',#2803,#2804,#1925,.T.);
#3469=EDGE_CURVE('',#2803,#2801,#1926,.T.);
#3470=EDGE_CURVE('',#2804,#2800,#1927,.T.);
#3471=EDGE_CURVE('',#2805,#2803,#1658,.T.);
#3472=EDGE_CURVE('',#2805,#2802,#1928,.T.);
#3473=EDGE_CURVE('',#2806,#2805,#1929,.T.);
#3474=EDGE_CURVE('',#2806,#2799,#1930,.T.);
#3475=EDGE_CURVE('',#2804,#2806,#1659,.F.);
#3476=EDGE_CURVE('',#2807,#2808,#1931,.T.);
#3477=EDGE_CURVE('',#2809,#2807,#1660,.T.);
#3478=EDGE_CURVE('',#2810,#2809,#1932,.F.);
#3479=EDGE_CURVE('',#2810,#2808,#1661,.T.);
#3480=EDGE_CURVE('',#2811,#2812,#1933,.F.);
#3481=EDGE_CURVE('',#2811,#2813,#1662,.T.);
#3482=EDGE_CURVE('',#2814,#2813,#1934,.T.);
#3483=EDGE_CURVE('',#2812,#2814,#1663,.T.);
#3484=EDGE_CURVE('',#2815,#2816,#1935,.F.);
#3485=EDGE_CURVE('',#2815,#2817,#1664,.T.);
#3486=EDGE_CURVE('',#2818,#2817,#1936,.T.);
#3487=EDGE_CURVE('',#2816,#2818,#1665,.T.);
#3488=EDGE_CURVE('',#2807,#2819,#1937,.T.);
#3489=EDGE_CURVE('',#2820,#2819,#1938,.T.);
#3490=EDGE_CURVE('',#2820,#2812,#1939,.T.);
#3491=EDGE_CURVE('',#2814,#2821,#1940,.T.);
#3492=EDGE_CURVE('',#2822,#2821,#1941,.T.);
#3493=EDGE_CURVE('',#2822,#2816,#1942,.T.);
#3494=EDGE_CURVE('',#2818,#2823,#1943,.T.);
#3495=EDGE_CURVE('',#2824,#2823,#1944,.T.);
#3496=EDGE_CURVE('',#2824,#2809,#1945,.T.);
#3497=EDGE_CURVE('',#2825,#2825,#1666,.F.);
#3498=EDGE_CURVE('',#2826,#2827,#1946,.T.);
#3499=EDGE_CURVE('',#2828,#2826,#1667,.T.);
#3500=EDGE_CURVE('',#2829,#2828,#1947,.F.);
#3501=EDGE_CURVE('',#2829,#2827,#1668,.T.);
#3502=EDGE_CURVE('',#2830,#2831,#1948,.F.);
#3503=EDGE_CURVE('',#2830,#2832,#1669,.T.);
#3504=EDGE_CURVE('',#2833,#2832,#1949,.T.);
#3505=EDGE_CURVE('',#2831,#2833,#1670,.T.);
#3506=EDGE_CURVE('',#2834,#2835,#1950,.F.);
#3507=EDGE_CURVE('',#2834,#2836,#1671,.T.);
#3508=EDGE_CURVE('',#2837,#2836,#1951,.T.);
#3509=EDGE_CURVE('',#2835,#2837,#1672,.T.);
#3510=EDGE_CURVE('',#2826,#2838,#1952,.T.);
#3511=EDGE_CURVE('',#2839,#2838,#1953,.T.);
#3512=EDGE_CURVE('',#2839,#2831,#1954,.T.);
#3513=EDGE_CURVE('',#2833,#2840,#1955,.T.);
#3514=EDGE_CURVE('',#2841,#2840,#1956,.T.);
#3515=EDGE_CURVE('',#2841,#2835,#1957,.T.);
#3516=EDGE_CURVE('',#2837,#2842,#1958,.T.);
#3517=EDGE_CURVE('',#2843,#2842,#1959,.T.);
#3518=EDGE_CURVE('',#2843,#2828,#1960,.T.);
#3519=EDGE_CURVE('',#2844,#2844,#1673,.F.);
#3520=EDGE_CURVE('',#2845,#2846,#1961,.T.);
#3521=EDGE_CURVE('',#2847,#2845,#1674,.T.);
#3522=EDGE_CURVE('',#2848,#2847,#1962,.F.);
#3523=EDGE_CURVE('',#2848,#2846,#1675,.T.);
#3524=EDGE_CURVE('',#2849,#2850,#1963,.F.);
#3525=EDGE_CURVE('',#2849,#2851,#1676,.T.);
#3526=EDGE_CURVE('',#2852,#2851,#1964,.T.);
#3527=EDGE_CURVE('',#2850,#2852,#1677,.T.);
#3528=EDGE_CURVE('',#2853,#2854,#1965,.F.);
#3529=EDGE_CURVE('',#2853,#2855,#1678,.T.);
#3530=EDGE_CURVE('',#2856,#2855,#1966,.T.);
#3531=EDGE_CURVE('',#2854,#2856,#1679,.T.);
#3532=EDGE_CURVE('',#2845,#2857,#1967,.T.);
#3533=EDGE_CURVE('',#2858,#2857,#1968,.T.);
#3534=EDGE_CURVE('',#2858,#2850,#1969,.T.);
#3535=EDGE_CURVE('',#2852,#2859,#1970,.T.);
#3536=EDGE_CURVE('',#2860,#2859,#1971,.T.);
#3537=EDGE_CURVE('',#2860,#2854,#1972,.T.);
#3538=EDGE_CURVE('',#2856,#2861,#1973,.T.);
#3539=EDGE_CURVE('',#2862,#2861,#1974,.T.);
#3540=EDGE_CURVE('',#2862,#2847,#1975,.T.);
#3541=EDGE_CURVE('',#2863,#2863,#1680,.F.);
#3542=EDGE_CURVE('',#2864,#2864,#1681,.T.);
#3543=EDGE_CURVE('',#2864,#2865,#1976,.T.);
#3544=EDGE_CURVE('',#2866,#2865,#395,.T.);
#3545=EDGE_CURVE('',#2867,#2866,#396,.T.);
#3546=EDGE_CURVE('',#2867,#2868,#1977,.T.);
#3547=EDGE_CURVE('',#2868,#2868,#1682,.T.);
#3548=EDGE_CURVE('',#2869,#2867,#397,.T.);
#3549=EDGE_CURVE('',#2865,#2869,#398,.T.);
#3550=EDGE_CURVE('',#2870,#2871,#399,.T.);
#3551=EDGE_CURVE('',#2871,#2870,#400,.T.);
#3552=EDGE_CURVE('',#2872,#2873,#401,.T.);
#3553=EDGE_CURVE('',#2873,#2872,#402,.T.);
#3554=EDGE_CURVE('',#2874,#2874,#1683,.T.);
#3555=EDGE_CURVE('',#2875,#2875,#1684,.T.);
#3556=EDGE_CURVE('',#2876,#2876,#1685,.T.);
#3557=EDGE_CURVE('',#2876,#2874,#1978,.T.);
#3558=EDGE_CURVE('',#2877,#2877,#1686,.T.);
#3559=EDGE_CURVE('',#2877,#2866,#1979,.T.);
#3560=EDGE_CURVE('',#2878,#2878,#1687,.T.);
#3561=EDGE_CURVE('',#2879,#2849,#1980,.T.);
#3562=EDGE_CURVE('',#2879,#2880,#1981,.T.);
#3563=EDGE_CURVE('',#2880,#2846,#1982,.T.);
#3564=EDGE_CURVE('',#2881,#2848,#1983,.T.);
#3565=EDGE_CURVE('',#2881,#2882,#1984,.T.);
#3566=EDGE_CURVE('',#2882,#2855,#1985,.T.);
#3567=EDGE_CURVE('',#2883,#2853,#1986,.T.);
#3568=EDGE_CURVE('',#2883,#2884,#1987,.T.);
#3569=EDGE_CURVE('',#2884,#2851,#1988,.T.);
#3570=EDGE_CURVE('',#2885,#2886,#1688,.T.);
#3571=EDGE_CURVE('',#2886,#2885,#1689,.T.);
#3572=EDGE_CURVE('',#2885,#2878,#1989,.T.);
#3573=EDGE_CURVE('',#2887,#2888,#403,.T.);
#3574=EDGE_CURVE('',#2889,#2887,#404,.T.);
#3575=EDGE_CURVE('',#2890,#2889,#405,.T.);
#3576=EDGE_CURVE('',#2890,#2863,#1990,.T.);
#3577=EDGE_CURVE('',#2888,#2890,#406,.T.);
#3578=EDGE_CURVE('',#2886,#2877,#1991,.T.);
#3579=EDGE_CURVE('',#2891,#2891,#1690,.T.);
#3580=EDGE_CURVE('',#2891,#2873,#1992,.T.);
#3581=EDGE_CURVE('',#2892,#2892,#1691,.T.);
#3582=EDGE_CURVE('',#2892,#2871,#1993,.T.);
#3583=EDGE_CURVE('',#2893,#2893,#1692,.T.);
#3584=EDGE_CURVE('',#2894,#2808,#1994,.T.);
#3585=EDGE_CURVE('',#2895,#2810,#1995,.T.);
#3586=EDGE_CURVE('',#2895,#2896,#1996,.T.);
#3587=EDGE_CURVE('',#2896,#2817,#1997,.T.);
#3588=EDGE_CURVE('',#2897,#2815,#1998,.T.);
#3589=EDGE_CURVE('',#2897,#2898,#1999,.T.);
#3590=EDGE_CURVE('',#2898,#2813,#2000,.T.);
#3591=EDGE_CURVE('',#2899,#2811,#2001,.T.);
#3592=EDGE_CURVE('',#2899,#2894,#2002,.T.);
#3593=EDGE_CURVE('',#2900,#2901,#1693,.T.);
#3594=EDGE_CURVE('',#2901,#2900,#1694,.T.);
#3595=EDGE_CURVE('',#2900,#2893,#2003,.T.);
#3596=EDGE_CURVE('',#2902,#2902,#1695,.T.);
#3597=EDGE_CURVE('',#2903,#2827,#2004,.T.);
#3598=EDGE_CURVE('',#2904,#2829,#2005,.T.);
#3599=EDGE_CURVE('',#2904,#2905,#2006,.T.);
#3600=EDGE_CURVE('',#2905,#2836,#2007,.T.);
#3601=EDGE_CURVE('',#2906,#2834,#2008,.T.);
#3602=EDGE_CURVE('',#2906,#2907,#2009,.T.);
#3603=EDGE_CURVE('',#2907,#2832,#2010,.T.);
#3604=EDGE_CURVE('',#2908,#2830,#2011,.T.);
#3605=EDGE_CURVE('',#2908,#2903,#2012,.T.);
#3606=EDGE_CURVE('',#2909,#2910,#1696,.T.);
#3607=EDGE_CURVE('',#2910,#2909,#1697,.T.);
#3608=EDGE_CURVE('',#2909,#2902,#2013,.T.);
#3609=EDGE_CURVE('',#2911,#2912,#407,.T.);
#3610=EDGE_CURVE('',#2912,#2911,#408,.T.);
#3611=EDGE_CURVE('',#2912,#2825,#2014,.T.);
#3612=EDGE_CURVE('',#2913,#2914,#409,.T.);
#3613=EDGE_CURVE('',#2914,#2913,#410,.T.);
#3614=EDGE_CURVE('',#2914,#2844,#2015,.T.);
#3615=EDGE_CURVE('',#2910,#2891,#2016,.T.);
#3616=EDGE_CURVE('',#2901,#2892,#2017,.T.);
#3617=EDGE_CURVE('',#2915,#2915,#1698,.F.);
#3618=EDGE_CURVE('',#2915,#2888,#2018,.T.);
#3619=EDGE_CURVE('',#2889,#2875,#2019,.T.);
#3620=EDGE_CURVE('',#2882,#2861,#2020,.T.);
#3621=EDGE_CURVE('',#2862,#2881,#2021,.T.);
#3622=EDGE_CURVE('',#2884,#2859,#2022,.T.);
#3623=EDGE_CURVE('',#2860,#2883,#2023,.T.);
#3624=EDGE_CURVE('',#2880,#2857,#2024,.T.);
#3625=EDGE_CURVE('',#2858,#2879,#2025,.T.);
#3626=EDGE_CURVE('',#2905,#2842,#2026,.T.);
#3627=EDGE_CURVE('',#2843,#2904,#2027,.T.);
#3628=EDGE_CURVE('',#2907,#2840,#2028,.T.);
#3629=EDGE_CURVE('',#2841,#2906,#2029,.T.);
#3630=EDGE_CURVE('',#2903,#2838,#2030,.T.);
#3631=EDGE_CURVE('',#2839,#2908,#2031,.T.);
#3632=EDGE_CURVE('',#2896,#2823,#2032,.T.);
#3633=EDGE_CURVE('',#2824,#2895,#2033,.T.);
#3634=EDGE_CURVE('',#2898,#2821,#2034,.T.);
#3635=EDGE_CURVE('',#2822,#2897,#2035,.T.);
#3636=EDGE_CURVE('',#2894,#2819,#2036,.T.);
#3637=EDGE_CURVE('',#2820,#2899,#2037,.T.);
#4585=ORIENTED_EDGE('',*,*,#3440,.T.);
#4586=ORIENTED_EDGE('',*,*,#3441,.T.);
#4587=ORIENTED_EDGE('',*,*,#3442,.T.);
#4588=ORIENTED_EDGE('',*,*,#3443,.T.);
#4589=ORIENTED_EDGE('',*,*,#3444,.F.);
#4590=ORIENTED_EDGE('',*,*,#3445,.T.);
#4591=ORIENTED_EDGE('',*,*,#3441,.F.);
#4592=ORIENTED_EDGE('',*,*,#3446,.F.);
#4593=ORIENTED_EDGE('',*,*,#3447,.F.);
#4594=ORIENTED_EDGE('',*,*,#3448,.T.);
#4595=ORIENTED_EDGE('',*,*,#3442,.F.);
#4596=ORIENTED_EDGE('',*,*,#3445,.F.);
#4597=ORIENTED_EDGE('',*,*,#3449,.F.);
#4598=ORIENTED_EDGE('',*,*,#3450,.T.);
#4599=ORIENTED_EDGE('',*,*,#3443,.F.);
#4600=ORIENTED_EDGE('',*,*,#3448,.F.);
#4601=ORIENTED_EDGE('',*,*,#3450,.F.);
#4602=ORIENTED_EDGE('',*,*,#3451,.F.);
#4603=ORIENTED_EDGE('',*,*,#3446,.T.);
#4604=ORIENTED_EDGE('',*,*,#3440,.F.);
#4605=ORIENTED_EDGE('',*,*,#3449,.T.);
#4606=ORIENTED_EDGE('',*,*,#3447,.T.);
#4607=ORIENTED_EDGE('',*,*,#3444,.T.);
#4608=ORIENTED_EDGE('',*,*,#3451,.T.);
#4609=ORIENTED_EDGE('',*,*,#3452,.T.);
#4610=ORIENTED_EDGE('',*,*,#3453,.T.);
#4611=ORIENTED_EDGE('',*,*,#3454,.T.);
#4612=ORIENTED_EDGE('',*,*,#3455,.T.);
#4613=ORIENTED_EDGE('',*,*,#3456,.F.);
#4614=ORIENTED_EDGE('',*,*,#3457,.T.);
#4615=ORIENTED_EDGE('',*,*,#3453,.F.);
#4616=ORIENTED_EDGE('',*,*,#3458,.F.);
#4617=ORIENTED_EDGE('',*,*,#3459,.F.);
#4618=ORIENTED_EDGE('',*,*,#3460,.T.);
#4619=ORIENTED_EDGE('',*,*,#3454,.F.);
#4620=ORIENTED_EDGE('',*,*,#3457,.F.);
#4621=ORIENTED_EDGE('',*,*,#3461,.F.);
#4622=ORIENTED_EDGE('',*,*,#3462,.T.);
#4623=ORIENTED_EDGE('',*,*,#3455,.F.);
#4624=ORIENTED_EDGE('',*,*,#3460,.F.);
#4625=ORIENTED_EDGE('',*,*,#3452,.F.);
#4626=ORIENTED_EDGE('',*,*,#3462,.F.);
#4627=ORIENTED_EDGE('',*,*,#3463,.F.);
#4628=ORIENTED_EDGE('',*,*,#3458,.T.);
#4629=ORIENTED_EDGE('',*,*,#3461,.T.);
#4630=ORIENTED_EDGE('',*,*,#3459,.T.);
#4631=ORIENTED_EDGE('',*,*,#3456,.T.);
#4632=ORIENTED_EDGE('',*,*,#3463,.T.);
#4633=ORIENTED_EDGE('',*,*,#3464,.T.);
#4634=ORIENTED_EDGE('',*,*,#3465,.T.);
#4635=ORIENTED_EDGE('',*,*,#3466,.T.);
#4636=ORIENTED_EDGE('',*,*,#3467,.T.);
#4637=ORIENTED_EDGE('',*,*,#3468,.F.);
#4638=ORIENTED_EDGE('',*,*,#3469,.T.);
#4639=ORIENTED_EDGE('',*,*,#3465,.F.);
#4640=ORIENTED_EDGE('',*,*,#3470,.F.);
#4641=ORIENTED_EDGE('',*,*,#3471,.F.);
#4642=ORIENTED_EDGE('',*,*,#3472,.T.);
#4643=ORIENTED_EDGE('',*,*,#3466,.F.);
#4644=ORIENTED_EDGE('',*,*,#3469,.F.);
#4645=ORIENTED_EDGE('',*,*,#3473,.F.);
#4646=ORIENTED_EDGE('',*,*,#3474,.T.);
#4647=ORIENTED_EDGE('',*,*,#3467,.F.);
#4648=ORIENTED_EDGE('',*,*,#3472,.F.);
#4649=ORIENTED_EDGE('',*,*,#3474,.F.);
#4650=ORIENTED_EDGE('',*,*,#3475,.F.);
#4651=ORIENTED_EDGE('',*,*,#3470,.T.);
#4652=ORIENTED_EDGE('',*,*,#3464,.F.);
#4653=ORIENTED_EDGE('',*,*,#3473,.T.);
#4654=ORIENTED_EDGE('',*,*,#3471,.T.);
#4655=ORIENTED_EDGE('',*,*,#3468,.T.);
#4656=ORIENTED_EDGE('',*,*,#3475,.T.);
#4657=ORIENTED_EDGE('',*,*,#3476,.F.);
#4658=ORIENTED_EDGE('',*,*,#3477,.F.);
#4659=ORIENTED_EDGE('',*,*,#3478,.F.);
#4660=ORIENTED_EDGE('',*,*,#3479,.T.);
#4661=ORIENTED_EDGE('',*,*,#3480,.F.);
#4662=ORIENTED_EDGE('',*,*,#3481,.T.);
#4663=ORIENTED_EDGE('',*,*,#3482,.F.);
#4664=ORIENTED_EDGE('',*,*,#3483,.F.);
#4665=ORIENTED_EDGE('',*,*,#3484,.F.);
#4666=ORIENTED_EDGE('',*,*,#3485,.T.);
#4667=ORIENTED_EDGE('',*,*,#3486,.F.);
#4668=ORIENTED_EDGE('',*,*,#3487,.F.);
#4669=ORIENTED_EDGE('',*,*,#3477,.T.);
#4670=ORIENTED_EDGE('',*,*,#3488,.T.);
#4671=ORIENTED_EDGE('',*,*,#3489,.F.);
#4672=ORIENTED_EDGE('',*,*,#3490,.T.);
#4673=ORIENTED_EDGE('',*,*,#3483,.T.);
#4674=ORIENTED_EDGE('',*,*,#3491,.T.);
#4675=ORIENTED_EDGE('',*,*,#3492,.F.);
#4676=ORIENTED_EDGE('',*,*,#3493,.T.);
#4677=ORIENTED_EDGE('',*,*,#3487,.T.);
#4678=ORIENTED_EDGE('',*,*,#3494,.T.);
#4679=ORIENTED_EDGE('',*,*,#3495,.F.);
#4680=ORIENTED_EDGE('',*,*,#3496,.T.);
#4681=ORIENTED_EDGE('',*,*,#3497,.T.);
#4682=ORIENTED_EDGE('',*,*,#3498,.F.);
#4683=ORIENTED_EDGE('',*,*,#3499,.F.);
#4684=ORIENTED_EDGE('',*,*,#3500,.F.);
#4685=ORIENTED_EDGE('',*,*,#3501,.T.);
#4686=ORIENTED_EDGE('',*,*,#3502,.F.);
#4687=ORIENTED_EDGE('',*,*,#3503,.T.);
#4688=ORIENTED_EDGE('',*,*,#3504,.F.);
#4689=ORIENTED_EDGE('',*,*,#3505,.F.);
#4690=ORIENTED_EDGE('',*,*,#3506,.F.);
#4691=ORIENTED_EDGE('',*,*,#3507,.T.);
#4692=ORIENTED_EDGE('',*,*,#3508,.F.);
#4693=ORIENTED_EDGE('',*,*,#3509,.F.);
#4694=ORIENTED_EDGE('',*,*,#3499,.T.);
#4695=ORIENTED_EDGE('',*,*,#3510,.T.);
#4696=ORIENTED_EDGE('',*,*,#3511,.F.);
#4697=ORIENTED_EDGE('',*,*,#3512,.T.);
#4698=ORIENTED_EDGE('',*,*,#3505,.T.);
#4699=ORIENTED_EDGE('',*,*,#3513,.T.);
#4700=ORIENTED_EDGE('',*,*,#3514,.F.);
#4701=ORIENTED_EDGE('',*,*,#3515,.T.);
#4702=ORIENTED_EDGE('',*,*,#3509,.T.);
#4703=ORIENTED_EDGE('',*,*,#3516,.T.);
#4704=ORIENTED_EDGE('',*,*,#3517,.F.);
#4705=ORIENTED_EDGE('',*,*,#3518,.T.);
#4706=ORIENTED_EDGE('',*,*,#3519,.T.);
#4707=ORIENTED_EDGE('',*,*,#3520,.F.);
#4708=ORIENTED_EDGE('',*,*,#3521,.F.);
#4709=ORIENTED_EDGE('',*,*,#3522,.F.);
#4710=ORIENTED_EDGE('',*,*,#3523,.T.);
#4711=ORIENTED_EDGE('',*,*,#3524,.F.);
#4712=ORIENTED_EDGE('',*,*,#3525,.T.);
#4713=ORIENTED_EDGE('',*,*,#3526,.F.);
#4714=ORIENTED_EDGE('',*,*,#3527,.F.);
#4715=ORIENTED_EDGE('',*,*,#3528,.F.);
#4716=ORIENTED_EDGE('',*,*,#3529,.T.);
#4717=ORIENTED_EDGE('',*,*,#3530,.F.);
#4718=ORIENTED_EDGE('',*,*,#3531,.F.);
#4719=ORIENTED_EDGE('',*,*,#3521,.T.);
#4720=ORIENTED_EDGE('',*,*,#3532,.T.);
#4721=ORIENTED_EDGE('',*,*,#3533,.F.);
#4722=ORIENTED_EDGE('',*,*,#3534,.T.);
#4723=ORIENTED_EDGE('',*,*,#3527,.T.);
#4724=ORIENTED_EDGE('',*,*,#3535,.T.);
#4725=ORIENTED_EDGE('',*,*,#3536,.F.);
#4726=ORIENTED_EDGE('',*,*,#3537,.T.);
#4727=ORIENTED_EDGE('',*,*,#3531,.T.);
#4728=ORIENTED_EDGE('',*,*,#3538,.T.);
#4729=ORIENTED_EDGE('',*,*,#3539,.F.);
#4730=ORIENTED_EDGE('',*,*,#3540,.T.);
#4731=ORIENTED_EDGE('',*,*,#3541,.T.);
#4732=ORIENTED_EDGE('',*,*,#3542,.T.);
#4733=ORIENTED_EDGE('',*,*,#3543,.T.);
#4734=ORIENTED_EDGE('',*,*,#3544,.F.);
#4735=ORIENTED_EDGE('',*,*,#3545,.F.);
#4736=ORIENTED_EDGE('',*,*,#3546,.T.);
#4737=ORIENTED_EDGE('',*,*,#3547,.F.);
#4738=ORIENTED_EDGE('',*,*,#3546,.F.);
#4739=ORIENTED_EDGE('',*,*,#3548,.F.);
#4740=ORIENTED_EDGE('',*,*,#3549,.F.);
#4741=ORIENTED_EDGE('',*,*,#3543,.F.);
#4742=ORIENTED_EDGE('',*,*,#3550,.F.);
#4743=ORIENTED_EDGE('',*,*,#3551,.F.);
#4744=ORIENTED_EDGE('',*,*,#3552,.F.);
#4745=ORIENTED_EDGE('',*,*,#3553,.F.);
#4746=ORIENTED_EDGE('',*,*,#3547,.T.);
#4747=ORIENTED_EDGE('',*,*,#3554,.F.);
#4748=ORIENTED_EDGE('',*,*,#3542,.F.);
#4749=ORIENTED_EDGE('',*,*,#3555,.F.);
#4750=ORIENTED_EDGE('',*,*,#3556,.F.);
#4751=ORIENTED_EDGE('',*,*,#3557,.T.);
#4752=ORIENTED_EDGE('',*,*,#3554,.T.);
#4753=ORIENTED_EDGE('',*,*,#3557,.F.);
#4754=ORIENTED_EDGE('',*,*,#3556,.T.);
#4755=ORIENTED_EDGE('',*,*,#3558,.F.);
#4756=ORIENTED_EDGE('',*,*,#3559,.T.);
#4757=ORIENTED_EDGE('',*,*,#3544,.T.);
#4758=ORIENTED_EDGE('',*,*,#3549,.T.);
#4759=ORIENTED_EDGE('',*,*,#3548,.T.);
#4760=ORIENTED_EDGE('',*,*,#3545,.T.);
#4761=ORIENTED_EDGE('',*,*,#3559,.F.);
#4762=ORIENTED_EDGE('',*,*,#3560,.T.);
#4763=ORIENTED_EDGE('',*,*,#3525,.F.);
#4764=ORIENTED_EDGE('',*,*,#3561,.F.);
#4765=ORIENTED_EDGE('',*,*,#3562,.T.);
#4766=ORIENTED_EDGE('',*,*,#3563,.T.);
#4767=ORIENTED_EDGE('',*,*,#3523,.F.);
#4768=ORIENTED_EDGE('',*,*,#3564,.F.);
#4769=ORIENTED_EDGE('',*,*,#3565,.T.);
#4770=ORIENTED_EDGE('',*,*,#3566,.T.);
#4771=ORIENTED_EDGE('',*,*,#3529,.F.);
#4772=ORIENTED_EDGE('',*,*,#3567,.F.);
#4773=ORIENTED_EDGE('',*,*,#3568,.T.);
#4774=ORIENTED_EDGE('',*,*,#3569,.T.);
#4775=ORIENTED_EDGE('',*,*,#3570,.T.);
#4776=ORIENTED_EDGE('',*,*,#3571,.T.);
#4777=ORIENTED_EDGE('',*,*,#3572,.T.);
#4778=ORIENTED_EDGE('',*,*,#3560,.F.);
#4779=ORIENTED_EDGE('',*,*,#3572,.F.);
#4780=ORIENTED_EDGE('',*,*,#3573,.F.);
#4781=ORIENTED_EDGE('',*,*,#3574,.F.);
#4782=ORIENTED_EDGE('',*,*,#3575,.F.);
#4783=ORIENTED_EDGE('',*,*,#3576,.T.);
#4784=ORIENTED_EDGE('',*,*,#3541,.F.);
#4785=ORIENTED_EDGE('',*,*,#3576,.F.);
#4786=ORIENTED_EDGE('',*,*,#3577,.F.);
#4787=ORIENTED_EDGE('',*,*,#3570,.F.);
#4788=ORIENTED_EDGE('',*,*,#3571,.F.);
#4789=ORIENTED_EDGE('',*,*,#3578,.T.);
#4790=ORIENTED_EDGE('',*,*,#3558,.T.);
#4791=ORIENTED_EDGE('',*,*,#3578,.F.);
#4792=ORIENTED_EDGE('',*,*,#3579,.F.);
#4793=ORIENTED_EDGE('',*,*,#3580,.T.);
#4794=ORIENTED_EDGE('',*,*,#3553,.T.);
#4795=ORIENTED_EDGE('',*,*,#3552,.T.);
#4796=ORIENTED_EDGE('',*,*,#3580,.F.);
#4797=ORIENTED_EDGE('',*,*,#3581,.F.);
#4798=ORIENTED_EDGE('',*,*,#3582,.T.);
#4799=ORIENTED_EDGE('',*,*,#3551,.T.);
#4800=ORIENTED_EDGE('',*,*,#3550,.T.);
#4801=ORIENTED_EDGE('',*,*,#3582,.F.);
#4802=ORIENTED_EDGE('',*,*,#3583,.T.);
#4803=ORIENTED_EDGE('',*,*,#3584,.T.);
#4804=ORIENTED_EDGE('',*,*,#3479,.F.);
#4805=ORIENTED_EDGE('',*,*,#3585,.F.);
#4806=ORIENTED_EDGE('',*,*,#3586,.T.);
#4807=ORIENTED_EDGE('',*,*,#3587,.T.);
#4808=ORIENTED_EDGE('',*,*,#3485,.F.);
#4809=ORIENTED_EDGE('',*,*,#3588,.F.);
#4810=ORIENTED_EDGE('',*,*,#3589,.T.);
#4811=ORIENTED_EDGE('',*,*,#3590,.T.);
#4812=ORIENTED_EDGE('',*,*,#3481,.F.);
#4813=ORIENTED_EDGE('',*,*,#3591,.F.);
#4814=ORIENTED_EDGE('',*,*,#3592,.T.);
#4815=ORIENTED_EDGE('',*,*,#3593,.T.);
#4816=ORIENTED_EDGE('',*,*,#3594,.T.);
#4817=ORIENTED_EDGE('',*,*,#3595,.T.);
#4818=ORIENTED_EDGE('',*,*,#3583,.F.);
#4819=ORIENTED_EDGE('',*,*,#3595,.F.);
#4820=ORIENTED_EDGE('',*,*,#3596,.T.);
#4821=ORIENTED_EDGE('',*,*,#3597,.T.);
#4822=ORIENTED_EDGE('',*,*,#3501,.F.);
#4823=ORIENTED_EDGE('',*,*,#3598,.F.);
#4824=ORIENTED_EDGE('',*,*,#3599,.T.);
#4825=ORIENTED_EDGE('',*,*,#3600,.T.);
#4826=ORIENTED_EDGE('',*,*,#3507,.F.);
#4827=ORIENTED_EDGE('',*,*,#3601,.F.);
#4828=ORIENTED_EDGE('',*,*,#3602,.T.);
#4829=ORIENTED_EDGE('',*,*,#3603,.T.);
#4830=ORIENTED_EDGE('',*,*,#3503,.F.);
#4831=ORIENTED_EDGE('',*,*,#3604,.F.);
#4832=ORIENTED_EDGE('',*,*,#3605,.T.);
#4833=ORIENTED_EDGE('',*,*,#3606,.T.);
#4834=ORIENTED_EDGE('',*,*,#3607,.T.);
#4835=ORIENTED_EDGE('',*,*,#3608,.T.);
#4836=ORIENTED_EDGE('',*,*,#3596,.F.);
#4837=ORIENTED_EDGE('',*,*,#3608,.F.);
#4838=ORIENTED_EDGE('',*,*,#3609,.F.);
#4839=ORIENTED_EDGE('',*,*,#3610,.F.);
#4840=ORIENTED_EDGE('',*,*,#3611,.T.);
#4841=ORIENTED_EDGE('',*,*,#3497,.F.);
#4842=ORIENTED_EDGE('',*,*,#3611,.F.);
#4843=ORIENTED_EDGE('',*,*,#3612,.F.);
#4844=ORIENTED_EDGE('',*,*,#3613,.F.);
#4845=ORIENTED_EDGE('',*,*,#3614,.T.);
#4846=ORIENTED_EDGE('',*,*,#3519,.F.);
#4847=ORIENTED_EDGE('',*,*,#3614,.F.);
#4848=ORIENTED_EDGE('',*,*,#3606,.F.);
#4849=ORIENTED_EDGE('',*,*,#3607,.F.);
#4850=ORIENTED_EDGE('',*,*,#3615,.T.);
#4851=ORIENTED_EDGE('',*,*,#3579,.T.);
#4852=ORIENTED_EDGE('',*,*,#3615,.F.);
#4853=ORIENTED_EDGE('',*,*,#3593,.F.);
#4854=ORIENTED_EDGE('',*,*,#3594,.F.);
#4855=ORIENTED_EDGE('',*,*,#3616,.T.);
#4856=ORIENTED_EDGE('',*,*,#3581,.T.);
#4857=ORIENTED_EDGE('',*,*,#3616,.F.);
#4858=ORIENTED_EDGE('',*,*,#3617,.T.);
#4859=ORIENTED_EDGE('',*,*,#3617,.F.);
#4860=ORIENTED_EDGE('',*,*,#3618,.T.);
#4861=ORIENTED_EDGE('',*,*,#3577,.T.);
#4862=ORIENTED_EDGE('',*,*,#3575,.T.);
#4863=ORIENTED_EDGE('',*,*,#3619,.T.);
#4864=ORIENTED_EDGE('',*,*,#3555,.T.);
#4865=ORIENTED_EDGE('',*,*,#3619,.F.);
#4866=ORIENTED_EDGE('',*,*,#3574,.T.);
#4867=ORIENTED_EDGE('',*,*,#3573,.T.);
#4868=ORIENTED_EDGE('',*,*,#3618,.F.);
#4869=ORIENTED_EDGE('',*,*,#3612,.T.);
#4870=ORIENTED_EDGE('',*,*,#3613,.T.);
#4871=ORIENTED_EDGE('',*,*,#3609,.T.);
#4872=ORIENTED_EDGE('',*,*,#3610,.T.);
#4873=ORIENTED_EDGE('',*,*,#3530,.T.);
#4874=ORIENTED_EDGE('',*,*,#3566,.F.);
#4875=ORIENTED_EDGE('',*,*,#3620,.T.);
#4876=ORIENTED_EDGE('',*,*,#3538,.F.);
#4877=ORIENTED_EDGE('',*,*,#3522,.T.);
#4878=ORIENTED_EDGE('',*,*,#3540,.F.);
#4879=ORIENTED_EDGE('',*,*,#3621,.T.);
#4880=ORIENTED_EDGE('',*,*,#3564,.T.);
#4881=ORIENTED_EDGE('',*,*,#3539,.T.);
#4882=ORIENTED_EDGE('',*,*,#3620,.F.);
#4883=ORIENTED_EDGE('',*,*,#3565,.F.);
#4884=ORIENTED_EDGE('',*,*,#3621,.F.);
#4885=ORIENTED_EDGE('',*,*,#3526,.T.);
#4886=ORIENTED_EDGE('',*,*,#3569,.F.);
#4887=ORIENTED_EDGE('',*,*,#3622,.T.);
#4888=ORIENTED_EDGE('',*,*,#3535,.F.);
#4889=ORIENTED_EDGE('',*,*,#3528,.T.);
#4890=ORIENTED_EDGE('',*,*,#3537,.F.);
#4891=ORIENTED_EDGE('',*,*,#3623,.T.);
#4892=ORIENTED_EDGE('',*,*,#3567,.T.);
#4893=ORIENTED_EDGE('',*,*,#3536,.T.);
#4894=ORIENTED_EDGE('',*,*,#3622,.F.);
#4895=ORIENTED_EDGE('',*,*,#3568,.F.);
#4896=ORIENTED_EDGE('',*,*,#3623,.F.);
#4897=ORIENTED_EDGE('',*,*,#3520,.T.);
#4898=ORIENTED_EDGE('',*,*,#3563,.F.);
#4899=ORIENTED_EDGE('',*,*,#3624,.T.);
#4900=ORIENTED_EDGE('',*,*,#3532,.F.);
#4901=ORIENTED_EDGE('',*,*,#3524,.T.);
#4902=ORIENTED_EDGE('',*,*,#3534,.F.);
#4903=ORIENTED_EDGE('',*,*,#3625,.T.);
#4904=ORIENTED_EDGE('',*,*,#3561,.T.);
#4905=ORIENTED_EDGE('',*,*,#3533,.T.);
#4906=ORIENTED_EDGE('',*,*,#3624,.F.);
#4907=ORIENTED_EDGE('',*,*,#3562,.F.);
#4908=ORIENTED_EDGE('',*,*,#3625,.F.);
#4909=ORIENTED_EDGE('',*,*,#3508,.T.);
#4910=ORIENTED_EDGE('',*,*,#3600,.F.);
#4911=ORIENTED_EDGE('',*,*,#3626,.T.);
#4912=ORIENTED_EDGE('',*,*,#3516,.F.);
#4913=ORIENTED_EDGE('',*,*,#3500,.T.);
#4914=ORIENTED_EDGE('',*,*,#3518,.F.);
#4915=ORIENTED_EDGE('',*,*,#3627,.T.);
#4916=ORIENTED_EDGE('',*,*,#3598,.T.);
#4917=ORIENTED_EDGE('',*,*,#3517,.T.);
#4918=ORIENTED_EDGE('',*,*,#3626,.F.);
#4919=ORIENTED_EDGE('',*,*,#3599,.F.);
#4920=ORIENTED_EDGE('',*,*,#3627,.F.);
#4921=ORIENTED_EDGE('',*,*,#3504,.T.);
#4922=ORIENTED_EDGE('',*,*,#3603,.F.);
#4923=ORIENTED_EDGE('',*,*,#3628,.T.);
#4924=ORIENTED_EDGE('',*,*,#3513,.F.);
#4925=ORIENTED_EDGE('',*,*,#3506,.T.);
#4926=ORIENTED_EDGE('',*,*,#3515,.F.);
#4927=ORIENTED_EDGE('',*,*,#3629,.T.);
#4928=ORIENTED_EDGE('',*,*,#3601,.T.);
#4929=ORIENTED_EDGE('',*,*,#3514,.T.);
#4930=ORIENTED_EDGE('',*,*,#3628,.F.);
#4931=ORIENTED_EDGE('',*,*,#3602,.F.);
#4932=ORIENTED_EDGE('',*,*,#3629,.F.);
#4933=ORIENTED_EDGE('',*,*,#3498,.T.);
#4934=ORIENTED_EDGE('',*,*,#3597,.F.);
#4935=ORIENTED_EDGE('',*,*,#3630,.T.);
#4936=ORIENTED_EDGE('',*,*,#3510,.F.);
#4937=ORIENTED_EDGE('',*,*,#3502,.T.);
#4938=ORIENTED_EDGE('',*,*,#3512,.F.);
#4939=ORIENTED_EDGE('',*,*,#3631,.T.);
#4940=ORIENTED_EDGE('',*,*,#3604,.T.);
#4941=ORIENTED_EDGE('',*,*,#3511,.T.);
#4942=ORIENTED_EDGE('',*,*,#3630,.F.);
#4943=ORIENTED_EDGE('',*,*,#3605,.F.);
#4944=ORIENTED_EDGE('',*,*,#3631,.F.);
#4945=ORIENTED_EDGE('',*,*,#3486,.T.);
#4946=ORIENTED_EDGE('',*,*,#3587,.F.);
#4947=ORIENTED_EDGE('',*,*,#3632,.T.);
#4948=ORIENTED_EDGE('',*,*,#3494,.F.);
#4949=ORIENTED_EDGE('',*,*,#3478,.T.);
#4950=ORIENTED_EDGE('',*,*,#3496,.F.);
#4951=ORIENTED_EDGE('',*,*,#3633,.T.);
#4952=ORIENTED_EDGE('',*,*,#3585,.T.);
#4953=ORIENTED_EDGE('',*,*,#3495,.T.);
#4954=ORIENTED_EDGE('',*,*,#3632,.F.);
#4955=ORIENTED_EDGE('',*,*,#3586,.F.);
#4956=ORIENTED_EDGE('',*,*,#3633,.F.);
#4957=ORIENTED_EDGE('',*,*,#3482,.T.);
#4958=ORIENTED_EDGE('',*,*,#3590,.F.);
#4959=ORIENTED_EDGE('',*,*,#3634,.T.);
#4960=ORIENTED_EDGE('',*,*,#3491,.F.);
#4961=ORIENTED_EDGE('',*,*,#3484,.T.);
#4962=ORIENTED_EDGE('',*,*,#3493,.F.);
#4963=ORIENTED_EDGE('',*,*,#3635,.T.);
#4964=ORIENTED_EDGE('',*,*,#3588,.T.);
#4965=ORIENTED_EDGE('',*,*,#3492,.T.);
#4966=ORIENTED_EDGE('',*,*,#3634,.F.);
#4967=ORIENTED_EDGE('',*,*,#3589,.F.);
#4968=ORIENTED_EDGE('',*,*,#3635,.F.);
#4969=ORIENTED_EDGE('',*,*,#3476,.T.);
#4970=ORIENTED_EDGE('',*,*,#3584,.F.);
#4971=ORIENTED_EDGE('',*,*,#3636,.T.);
#4972=ORIENTED_EDGE('',*,*,#3488,.F.);
#4973=ORIENTED_EDGE('',*,*,#3480,.T.);
#4974=ORIENTED_EDGE('',*,*,#3490,.F.);
#4975=ORIENTED_EDGE('',*,*,#3637,.T.);
#4976=ORIENTED_EDGE('',*,*,#3591,.T.);
#4977=ORIENTED_EDGE('',*,*,#3489,.T.);
#4978=ORIENTED_EDGE('',*,*,#3636,.F.);
#4979=ORIENTED_EDGE('',*,*,#3592,.F.);
#4980=ORIENTED_EDGE('',*,*,#3637,.F.);
#5667=PLANE('',#6479);
#5668=PLANE('',#6482);
#5669=PLANE('',#6485);
#5670=PLANE('',#6488);
#5671=PLANE('',#6489);
#5672=PLANE('',#6492);
#5673=PLANE('',#6495);
#5674=PLANE('',#6498);
#5675=PLANE('',#6499);
#5676=PLANE('',#6502);
#5677=PLANE('',#6505);
#5678=PLANE('',#6508);
#5679=PLANE('',#6518);
#5680=PLANE('',#6529);
#5681=PLANE('',#6540);
#5682=PLANE('',#6545);
#5683=PLANE('',#6547);
#5684=PLANE('',#6551);
#5685=PLANE('',#6554);
#5686=PLANE('',#6565);
#5687=PLANE('',#6570);
#5688=PLANE('',#6579);
#5689=PLANE('',#6582);
#5690=PLANE('',#6583);
#5691=PLANE('',#6584);
#5692=PLANE('',#6585);
#5693=PLANE('',#6586);
#5694=PLANE('',#6587);
#5695=PLANE('',#6588);
#5696=PLANE('',#6589);
#5697=PLANE('',#6590);
#5698=PLANE('',#6591);
#5699=PLANE('',#6592);
#5700=PLANE('',#6593);
#5701=PLANE('',#6594);
#5702=PLANE('',#6595);
#5703=PLANE('',#6596);
#5704=PLANE('',#6597);
#5705=PLANE('',#6598);
#5706=PLANE('',#6599);
#5707=PLANE('',#6600);
#5708=PLANE('',#6601);
#5709=PLANE('',#6602);
#5710=PLANE('',#6603);
#5711=PLANE('',#6604);
#5712=PLANE('',#6605);
#5713=PLANE('',#6606);
#5714=PLANE('',#6607);
#5715=PLANE('',#6608);
#5909=ADVANCED_FACE('',(#860),#5667,.T.);
#5910=ADVANCED_FACE('',(#861),#5668,.T.);
#5911=ADVANCED_FACE('',(#862),#527,.F.);
#5912=ADVANCED_FACE('',(#863),#5669,.T.);
#5913=ADVANCED_FACE('',(#864),#528,.T.);
#5914=ADVANCED_FACE('',(#865),#5670,.F.);
#5915=ADVANCED_FACE('',(#866),#5671,.T.);
#5916=ADVANCED_FACE('',(#867),#5672,.T.);
#5917=ADVANCED_FACE('',(#868),#529,.F.);
#5918=ADVANCED_FACE('',(#869),#5673,.T.);
#5919=ADVANCED_FACE('',(#870),#530,.T.);
#5920=ADVANCED_FACE('',(#871),#5674,.F.);
#5921=ADVANCED_FACE('',(#872),#5675,.T.);
#5922=ADVANCED_FACE('',(#873),#5676,.T.);
#5923=ADVANCED_FACE('',(#874),#531,.F.);
#5924=ADVANCED_FACE('',(#875),#5677,.T.);
#5925=ADVANCED_FACE('',(#876),#532,.T.);
#5926=ADVANCED_FACE('',(#877),#5678,.F.);
#5927=ADVANCED_FACE('',(#878),#533,.T.);
#5928=ADVANCED_FACE('',(#879),#534,.T.);
#5929=ADVANCED_FACE('',(#880),#535,.T.);
#5930=ADVANCED_FACE('',(#881,#663),#5679,.T.);
#5931=ADVANCED_FACE('',(#882),#536,.T.);
#5932=ADVANCED_FACE('',(#883),#537,.T.);
#5933=ADVANCED_FACE('',(#884),#538,.T.);
#5934=ADVANCED_FACE('',(#885,#664),#5680,.T.);
#5935=ADVANCED_FACE('',(#886),#539,.T.);
#5936=ADVANCED_FACE('',(#887),#540,.T.);
#5937=ADVANCED_FACE('',(#888),#541,.T.);
#5938=ADVANCED_FACE('',(#889,#665),#5681,.T.);
#5939=ADVANCED_FACE('',(#890,#666,#667),#542,.T.);
#5940=ADVANCED_FACE('',(#891,#668),#5682,.T.);
#5941=ADVANCED_FACE('',(#892,#669),#5683,.F.);
#5942=ADVANCED_FACE('',(#893),#543,.F.);
#5943=ADVANCED_FACE('',(#894),#5684,.T.);
#5944=ADVANCED_FACE('',(#895),#544,.T.);
#5945=ADVANCED_FACE('',(#896,#670),#5685,.T.);
#5946=ADVANCED_FACE('',(#897),#545,.T.);
#5947=ADVANCED_FACE('',(#898),#546,.F.);
#5948=ADVANCED_FACE('',(#899),#191,.T.);
#5949=ADVANCED_FACE('',(#900),#547,.T.);
#5950=ADVANCED_FACE('',(#901),#548,.T.);
#5951=ADVANCED_FACE('',(#902,#671),#5686,.T.);
#5952=ADVANCED_FACE('',(#903),#549,.T.);
#5953=ADVANCED_FACE('',(#904,#672),#5687,.T.);
#5954=ADVANCED_FACE('',(#905),#550,.T.);
#5955=ADVANCED_FACE('',(#906),#551,.F.);
#5956=ADVANCED_FACE('',(#907),#552,.F.);
#5957=ADVANCED_FACE('',(#908),#192,.T.);
#5958=ADVANCED_FACE('',(#909),#193,.T.);
#5959=ADVANCED_FACE('',(#910),#5688,.F.);
#5960=ADVANCED_FACE('',(#911,#673,#674),#553,.F.);
#5961=ADVANCED_FACE('',(#912),#5689,.T.);
#5962=ADVANCED_FACE('',(#913),#5690,.T.);
#5963=ADVANCED_FACE('',(#914),#5691,.F.);
#5964=ADVANCED_FACE('',(#915),#5692,.T.);
#5965=ADVANCED_FACE('',(#916),#5693,.T.);
#5966=ADVANCED_FACE('',(#917),#5694,.F.);
#5967=ADVANCED_FACE('',(#918),#5695,.T.);
#5968=ADVANCED_FACE('',(#919),#5696,.T.);
#5969=ADVANCED_FACE('',(#920),#5697,.F.);
#5970=ADVANCED_FACE('',(#921),#5698,.T.);
#5971=ADVANCED_FACE('',(#922),#5699,.T.);
#5972=ADVANCED_FACE('',(#923),#5700,.F.);
#5973=ADVANCED_FACE('',(#924),#5701,.T.);
#5974=ADVANCED_FACE('',(#925),#5702,.T.);
#5975=ADVANCED_FACE('',(#926),#5703,.F.);
#5976=ADVANCED_FACE('',(#927),#5704,.T.);
#5977=ADVANCED_FACE('',(#928),#5705,.T.);
#5978=ADVANCED_FACE('',(#929),#5706,.F.);
#5979=ADVANCED_FACE('',(#930),#5707,.T.);
#5980=ADVANCED_FACE('',(#931),#5708,.T.);
#5981=ADVANCED_FACE('',(#932),#5709,.F.);
#5982=ADVANCED_FACE('',(#933),#5710,.T.);
#5983=ADVANCED_FACE('',(#934),#5711,.T.);
#5984=ADVANCED_FACE('',(#935),#5712,.F.);
#5985=ADVANCED_FACE('',(#936),#5713,.T.);
#5986=ADVANCED_FACE('',(#937),#5714,.T.);
#5987=ADVANCED_FACE('',(#938),#5715,.F.);
#6137=CLOSED_SHELL('',(#5909,#5910,#5911,#5912,#5913,#5914));
#6138=CLOSED_SHELL('',(#5915,#5916,#5917,#5918,#5919,#5920));
#6139=CLOSED_SHELL('',(#5921,#5922,#5923,#5924,#5925,#5926));
#6140=CLOSED_SHELL('',(#5927,#5928,#5929,#5930,#5931,#5932,#5933,#5934,
#5935,#5936,#5937,#5938,#5939,#5940,#5941,#5942,#5943,#5944,#5945,#5946,
#5947,#5948,#5949,#5950,#5951,#5952,#5953,#5954,#5955,#5956,#5957,#5958,
#5959,#5960,#5961,#5962,#5963,#5964,#5965,#5966,#5967,#5968,#5969,#5970,
#5971,#5972,#5973,#5974,#5975,#5976,#5977,#5978,#5979,#5980,#5981,#5982,
#5983,#5984,#5985,#5986,#5987));
#6478=AXIS2_PLACEMENT_3D('',#11498,#7451,#7452);
#6479=AXIS2_PLACEMENT_3D('',#11499,#7453,#7454);
#6480=AXIS2_PLACEMENT_3D('',#11502,#7455,#7456);
#6481=AXIS2_PLACEMENT_3D('',#11506,#7458,#7459);
#6482=AXIS2_PLACEMENT_3D('',#11508,#7461,#7462);
#6483=AXIS2_PLACEMENT_3D('',#11514,#7466,#7467);
#6484=AXIS2_PLACEMENT_3D('',#11516,#7468,#7469);
#6485=AXIS2_PLACEMENT_3D('',#11518,#7471,#7472);
#6486=AXIS2_PLACEMENT_3D('',#11522,#7475,#7476);
#6487=AXIS2_PLACEMENT_3D('',#11523,#7477,#7478);
#6488=AXIS2_PLACEMENT_3D('',#11524,#7479,#7480);
#6489=AXIS2_PLACEMENT_3D('',#11525,#7481,#7482);
#6490=AXIS2_PLACEMENT_3D('',#11528,#7483,#7484);
#6491=AXIS2_PLACEMENT_3D('',#11532,#7486,#7487);
#6492=AXIS2_PLACEMENT_3D('',#11534,#7489,#7490);
#6493=AXIS2_PLACEMENT_3D('',#11540,#7494,#7495);
#6494=AXIS2_PLACEMENT_3D('',#11542,#7496,#7497);
#6495=AXIS2_PLACEMENT_3D('',#11544,#7499,#7500);
#6496=AXIS2_PLACEMENT_3D('',#11548,#7503,#7504);
#6497=AXIS2_PLACEMENT_3D('',#11549,#7505,#7506);
#6498=AXIS2_PLACEMENT_3D('',#11550,#7507,#7508);
#6499=AXIS2_PLACEMENT_3D('',#11551,#7509,#7510);
#6500=AXIS2_PLACEMENT_3D('',#11554,#7511,#7512);
#6501=AXIS2_PLACEMENT_3D('',#11558,#7514,#7515);
#6502=AXIS2_PLACEMENT_3D('',#11560,#7517,#7518);
#6503=AXIS2_PLACEMENT_3D('',#11566,#7522,#7523);
#6504=AXIS2_PLACEMENT_3D('',#11568,#7524,#7525);
#6505=AXIS2_PLACEMENT_3D('',#11570,#7527,#7528);
#6506=AXIS2_PLACEMENT_3D('',#11574,#7531,#7532);
#6507=AXIS2_PLACEMENT_3D('',#11575,#7533,#7534);
#6508=AXIS2_PLACEMENT_3D('',#11576,#7535,#7536);
#6509=AXIS2_PLACEMENT_3D('',#11577,#7537,#7538);
#6510=AXIS2_PLACEMENT_3D('',#11582,#7540,#7541);
#6511=AXIS2_PLACEMENT_3D('',#11585,#7543,#7544);
#6512=AXIS2_PLACEMENT_3D('',#11586,#7545,#7546);
#6513=AXIS2_PLACEMENT_3D('',#11591,#7548,#7549);
#6514=AXIS2_PLACEMENT_3D('',#11594,#7551,#7552);
#6515=AXIS2_PLACEMENT_3D('',#11595,#7553,#7554);
#6516=AXIS2_PLACEMENT_3D('',#11600,#7556,#7557);
#6517=AXIS2_PLACEMENT_3D('',#11603,#7559,#7560);
#6518=AXIS2_PLACEMENT_3D('',#11604,#7561,#7562);
#6519=AXIS2_PLACEMENT_3D('',#11621,#7572,#7573);
#6520=AXIS2_PLACEMENT_3D('',#11622,#7574,#7575);
#6521=AXIS2_PLACEMENT_3D('',#11627,#7577,#7578);
#6522=AXIS2_PLACEMENT_3D('',#11630,#7580,#7581);
#6523=AXIS2_PLACEMENT_3D('',#11631,#7582,#7583);
#6524=AXIS2_PLACEMENT_3D('',#11636,#7585,#7586);
#6525=AXIS2_PLACEMENT_3D('',#11639,#7588,#7589);
#6526=AXIS2_PLACEMENT_3D('',#11640,#7590,#7591);
#6527=AXIS2_PLACEMENT_3D('',#11645,#7593,#7594);
#6528=AXIS2_PLACEMENT_3D('',#11648,#7596,#7597);
#6529=AXIS2_PLACEMENT_3D('',#11649,#7598,#7599);
#6530=AXIS2_PLACEMENT_3D('',#11666,#7609,#7610);
#6531=AXIS2_PLACEMENT_3D('',#11667,#7611,#7612);
#6532=AXIS2_PLACEMENT_3D('',#11672,#7614,#7615);
#6533=AXIS2_PLACEMENT_3D('',#11675,#7617,#7618);
#6534=AXIS2_PLACEMENT_3D('',#11676,#7619,#7620);
#6535=AXIS2_PLACEMENT_3D('',#11681,#7622,#7623);
#6536=AXIS2_PLACEMENT_3D('',#11684,#7625,#7626);
#6537=AXIS2_PLACEMENT_3D('',#11685,#7627,#7628);
#6538=AXIS2_PLACEMENT_3D('',#11690,#7630,#7631);
#6539=AXIS2_PLACEMENT_3D('',#11693,#7633,#7634);
#6540=AXIS2_PLACEMENT_3D('',#11694,#7635,#7636);
#6541=AXIS2_PLACEMENT_3D('',#11711,#7646,#7647);
#6542=AXIS2_PLACEMENT_3D('',#11712,#7648,#7649);
#6543=AXIS2_PLACEMENT_3D('',#11714,#7650,#7651);
#6544=AXIS2_PLACEMENT_3D('',#11749,#7654,#7655);
#6545=AXIS2_PLACEMENT_3D('',#11887,#7656,#7657);
#6546=AXIS2_PLACEMENT_3D('',#11889,#7658,#7659);
#6547=AXIS2_PLACEMENT_3D('',#11890,#7660,#7661);
#6548=AXIS2_PLACEMENT_3D('',#11892,#7662,#7663);
#6549=AXIS2_PLACEMENT_3D('',#11893,#7664,#7665);
#6550=AXIS2_PLACEMENT_3D('',#11895,#7666,#7667);
#6551=AXIS2_PLACEMENT_3D('',#11897,#7669,#7670);
#6552=AXIS2_PLACEMENT_3D('',#11898,#7671,#7672);
#6553=AXIS2_PLACEMENT_3D('',#11900,#7673,#7674);
#6554=AXIS2_PLACEMENT_3D('',#11902,#7676,#7677);
#6555=AXIS2_PLACEMENT_3D('',#11904,#7678,#7679);
#6556=AXIS2_PLACEMENT_3D('',#11920,#7689,#7690);
#6557=AXIS2_PLACEMENT_3D('',#11923,#7691,#7692);
#6558=AXIS2_PLACEMENT_3D('',#11924,#7693,#7694);
#6559=AXIS2_PLACEMENT_3D('',#11926,#7696,#7697);
#6560=AXIS2_PLACEMENT_3D('',#11988,#7699,#7700);
#6561=AXIS2_PLACEMENT_3D('',#11990,#7702,#7703);
#6562=AXIS2_PLACEMENT_3D('',#11992,#7704,#7705);
#6563=AXIS2_PLACEMENT_3D('',#11994,#7707,#7708);
#6564=AXIS2_PLACEMENT_3D('',#11996,#7709,#7710);
#6565=AXIS2_PLACEMENT_3D('',#11998,#7712,#7713);
#6566=AXIS2_PLACEMENT_3D('',#12000,#7714,#7715);
#6567=AXIS2_PLACEMENT_3D('',#12016,#7725,#7726);
#6568=AXIS2_PLACEMENT_3D('',#12019,#7727,#7728);
#6569=AXIS2_PLACEMENT_3D('',#12020,#7729,#7730);
#6570=AXIS2_PLACEMENT_3D('',#12022,#7732,#7733);
#6571=AXIS2_PLACEMENT_3D('',#12024,#7734,#7735);
#6572=AXIS2_PLACEMENT_3D('',#12040,#7745,#7746);
#6573=AXIS2_PLACEMENT_3D('',#12043,#7747,#7748);
#6574=AXIS2_PLACEMENT_3D('',#12044,#7749,#7750);
#6575=AXIS2_PLACEMENT_3D('',#12046,#7752,#7753);
#6576=AXIS2_PLACEMENT_3D('',#12102,#7755,#7756);
#6577=AXIS2_PLACEMENT_3D('',#12158,#7758,#7759);
#6578=AXIS2_PLACEMENT_3D('',#12160,#7761,#7762);
#6579=AXIS2_PLACEMENT_3D('',#12162,#7764,#7765);
#6580=AXIS2_PLACEMENT_3D('',#12164,#7766,#7767);
#6581=AXIS2_PLACEMENT_3D('',#12165,#7768,#7769);
#6582=AXIS2_PLACEMENT_3D('',#12168,#7772,#7773);
#6583=AXIS2_PLACEMENT_3D('',#12170,#7775,#7776);
#6584=AXIS2_PLACEMENT_3D('',#12172,#7778,#7779);
#6585=AXIS2_PLACEMENT_3D('',#12173,#7780,#7781);
#6586=AXIS2_PLACEMENT_3D('',#12175,#7783,#7784);
#6587=AXIS2_PLACEMENT_3D('',#12177,#7786,#7787);
#6588=AXIS2_PLACEMENT_3D('',#12178,#7788,#7789);
#6589=AXIS2_PLACEMENT_3D('',#12180,#7791,#7792);
#6590=AXIS2_PLACEMENT_3D('',#12182,#7794,#7795);
#6591=AXIS2_PLACEMENT_3D('',#12183,#7796,#7797);
#6592=AXIS2_PLACEMENT_3D('',#12185,#7799,#7800);
#6593=AXIS2_PLACEMENT_3D('',#12187,#7802,#7803);
#6594=AXIS2_PLACEMENT_3D('',#12188,#7804,#7805);
#6595=AXIS2_PLACEMENT_3D('',#12190,#7807,#7808);
#6596=AXIS2_PLACEMENT_3D('',#12192,#7810,#7811);
#6597=AXIS2_PLACEMENT_3D('',#12193,#7812,#7813);
#6598=AXIS2_PLACEMENT_3D('',#12195,#7815,#7816);
#6599=AXIS2_PLACEMENT_3D('',#12197,#7818,#7819);
#6600=AXIS2_PLACEMENT_3D('',#12198,#7820,#7821);
#6601=AXIS2_PLACEMENT_3D('',#12200,#7823,#7824);
#6602=AXIS2_PLACEMENT_3D('',#12202,#7826,#7827);
#6603=AXIS2_PLACEMENT_3D('',#12203,#7828,#7829);
#6604=AXIS2_PLACEMENT_3D('',#12205,#7831,#7832);
#6605=AXIS2_PLACEMENT_3D('',#12207,#7834,#7835);
#6606=AXIS2_PLACEMENT_3D('',#12208,#7836,#7837);
#6607=AXIS2_PLACEMENT_3D('',#12210,#7839,#7840);
#6608=AXIS2_PLACEMENT_3D('',#12212,#7842,#7843);
#7451=DIRECTION('axis',(0.,0.,1.));
#7452=DIRECTION('refdir',(1.,0.,0.));
#7453=DIRECTION('center_axis',(1.3988810110277E-14,0.,1.));
#7454=DIRECTION('ref_axis',(1.,0.,-1.3988810110277E-14));
#7455=DIRECTION('center_axis',(1.3988810110277E-14,0.,1.));
#7456=DIRECTION('ref_axis',(1.,0.,-1.3988810110277E-14));
#7457=DIRECTION('',(-0.86602540378444,-0.499999999999998,8.88178419698879E-15));
#7458=DIRECTION('center_axis',(-1.3988810110277E-14,0.,-1.));
#7459=DIRECTION('ref_axis',(1.,0.,-1.3988810110277E-14));
#7460=DIRECTION('',(-0.866025403784435,-0.500000000000007,1.77635683939776E-14));
#7461=DIRECTION('center_axis',(-0.499999999999999,0.866025403784439,6.99440505513849E-15));
#7462=DIRECTION('ref_axis',(0.,-8.07644328281097E-15,1.));
#7463=DIRECTION('',(0.866025403784439,0.499999999999999,0.));
#7464=DIRECTION('',(1.39967402747386E-14,0.,1.));
#7465=DIRECTION('',(1.39967402747386E-14,0.,1.));
#7466=DIRECTION('center_axis',(1.3988810110277E-14,0.,1.));
#7467=DIRECTION('ref_axis',(1.,0.,-1.3988810110277E-14));
#7468=DIRECTION('center_axis',(0.,0.,1.));
#7469=DIRECTION('ref_axis',(1.,0.,0.));
#7470=DIRECTION('',(1.39967402747385E-14,0.,1.));
#7471=DIRECTION('center_axis',(-0.500000000000006,0.866025403784435,6.96664947952286E-15));
#7472=DIRECTION('ref_axis',(1.39332989590456E-14,0.,1.));
#7473=DIRECTION('',(0.866025403784434,0.500000000000008,0.));
#7474=DIRECTION('',(1.39967402747385E-14,0.,1.));
#7475=DIRECTION('center_axis',(1.3988810110277E-14,0.,1.));
#7476=DIRECTION('ref_axis',(1.,0.,-1.3988810110277E-14));
#7477=DIRECTION('center_axis',(0.,0.,1.));
#7478=DIRECTION('ref_axis',(1.,0.,0.));
#7479=DIRECTION('center_axis',(0.,0.,1.));
#7480=DIRECTION('ref_axis',(1.,0.,0.));
#7481=DIRECTION('center_axis',(-0.866025403784443,0.,-0.499999999999992));
#7482=DIRECTION('ref_axis',(-0.499999999999992,0.,0.866025403784443));
#7483=DIRECTION('center_axis',(-0.866025403784443,0.,-0.499999999999992));
#7484=DIRECTION('ref_axis',(-0.499999999999992,0.,0.866025403784443));
#7485=DIRECTION('',(0.433012701892206,-0.5,-0.750000000000008));
#7486=DIRECTION('center_axis',(0.866025403784443,0.,0.499999999999992));
#7487=DIRECTION('ref_axis',(-0.499999999999992,0.,0.866025403784443));
#7488=DIRECTION('',(0.433012701892208,-0.500000000000003,-0.750000000000004));
#7489=DIRECTION('center_axis',(0.249999999999996,0.866025403784439,-0.433012701892221));
#7490=DIRECTION('ref_axis',(0.,0.447213595499959,0.894427190999915));
#7491=DIRECTION('',(-0.433012701892213,0.499999999999998,0.750000000000005));
#7492=DIRECTION('',(-0.866025403784443,0.,-0.499999999999992));
#7493=DIRECTION('',(-0.866025403784443,0.,-0.499999999999992));
#7494=DIRECTION('center_axis',(-0.866025403784443,0.,-0.499999999999992));
#7495=DIRECTION('ref_axis',(-0.499999999999992,0.,0.866025403784443));
#7496=DIRECTION('center_axis',(-0.866025403784443,0.,-0.499999999999992));
#7497=DIRECTION('ref_axis',(-0.499999999999992,0.,0.866025403784443));
#7498=DIRECTION('',(-0.866025403784443,0.,-0.499999999999992));
#7499=DIRECTION('center_axis',(0.249999999999999,0.866025403784435,-0.433012701892227));
#7500=DIRECTION('ref_axis',(-0.866025403784443,0.,-0.499999999999992));
#7501=DIRECTION('',(-0.433012701892207,0.50000000000001,0.750000000000001));
#7502=DIRECTION('',(-0.866025403784443,0.,-0.499999999999992));
#7503=DIRECTION('center_axis',(-0.866025403784443,0.,-0.499999999999992));
#7504=DIRECTION('ref_axis',(-0.499999999999992,0.,0.866025403784443));
#7505=DIRECTION('center_axis',(-0.866025403784443,0.,-0.499999999999992));
#7506=DIRECTION('ref_axis',(-0.499999999999992,0.,0.866025403784443));
#7507=DIRECTION('center_axis',(-0.866025403784443,0.,-0.499999999999992));
#7508=DIRECTION('ref_axis',(-0.499999999999992,0.,0.866025403784443));
#7509=DIRECTION('center_axis',(0.866025403784429,0.,-0.500000000000016));
#7510=DIRECTION('ref_axis',(-0.500000000000016,0.,-0.866025403784429));
#7511=DIRECTION('center_axis',(0.866025403784429,0.,-0.500000000000016));
#7512=DIRECTION('ref_axis',(-0.500000000000016,0.,-0.866025403784429));
#7513=DIRECTION('',(0.433012701892233,-0.5,0.749999999999992));
#7514=DIRECTION('center_axis',(-0.866025403784429,0.,0.500000000000016));
#7515=DIRECTION('ref_axis',(-0.500000000000016,0.,-0.866025403784429));
#7516=DIRECTION('',(0.433012701892229,-0.500000000000006,0.749999999999991));
#7517=DIRECTION('center_axis',(0.250000000000008,0.866025403784439,0.433012701892214));
#7518=DIRECTION('ref_axis',(0.,-0.447213595499953,0.894427190999918));
#7519=DIRECTION('',(-0.433012701892223,0.500000000000001,-0.749999999999997));
#7520=DIRECTION('',(0.866025403784429,0.,-0.500000000000016));
#7521=DIRECTION('',(0.866025403784429,0.,-0.500000000000016));
#7522=DIRECTION('center_axis',(0.866025403784429,0.,-0.500000000000016));
#7523=DIRECTION('ref_axis',(-0.500000000000016,0.,-0.866025403784429));
#7524=DIRECTION('center_axis',(0.866025403784436,0.,-0.500000000000004));
#7525=DIRECTION('ref_axis',(-0.500000000000004,0.,-0.866025403784436));
#7526=DIRECTION('',(0.866025403784429,0.,-0.500000000000016));
#7527=DIRECTION('center_axis',(0.250000000000011,0.866025403784435,0.43301270189222));
#7528=DIRECTION('ref_axis',(0.866025403784429,0.,-0.500000000000016));
#7529=DIRECTION('',(-0.433012701892228,0.500000000000006,-0.749999999999991));
#7530=DIRECTION('',(0.866025403784429,0.,-0.500000000000016));
#7531=DIRECTION('center_axis',(0.866025403784429,0.,-0.500000000000016));
#7532=DIRECTION('ref_axis',(-0.500000000000016,0.,-0.866025403784429));
#7533=DIRECTION('center_axis',(0.866025403784436,0.,-0.500000000000004));
#7534=DIRECTION('ref_axis',(-0.500000000000004,0.,-0.866025403784436));
#7535=DIRECTION('center_axis',(0.866025403784436,0.,-0.500000000000004));
#7536=DIRECTION('ref_axis',(-0.500000000000004,0.,-0.866025403784436));
#7537=DIRECTION('center_axis',(0.866025403784443,0.,0.499999999999992));
#7538=DIRECTION('ref_axis',(-0.321393804843261,0.766044443118984,0.556670399226416));
#7539=DIRECTION('',(0.866025403784442,0.,0.499999999999994));
#7540=DIRECTION('center_axis',(-0.866025403784443,0.,-0.499999999999992));
#7541=DIRECTION('ref_axis',(-0.499999999999992,0.,0.866025403784443));
#7542=DIRECTION('',(0.866025403784443,0.,0.499999999999992));
#7543=DIRECTION('center_axis',(-0.866025403784443,0.,-0.499999999999992));
#7544=DIRECTION('ref_axis',(-0.499999999999992,0.,0.866025403784443));
#7545=DIRECTION('center_axis',(0.866025403784443,0.,0.499999999999992));
#7546=DIRECTION('ref_axis',(0.499999999999992,0.,-0.866025403784443));
#7547=DIRECTION('',(0.866025403784443,0.,0.499999999999992));
#7548=DIRECTION('center_axis',(-0.866025403784443,0.,-0.499999999999992));
#7549=DIRECTION('ref_axis',(-0.499999999999992,0.,0.866025403784443));
#7550=DIRECTION('',(0.866025403784443,0.,0.499999999999992));
#7551=DIRECTION('center_axis',(-0.866025403784443,0.,-0.499999999999992));
#7552=DIRECTION('ref_axis',(-0.499999999999992,0.,0.866025403784443));
#7553=DIRECTION('center_axis',(0.866025403784443,0.,0.499999999999992));
#7554=DIRECTION('ref_axis',(0.499999999999992,0.,-0.866025403784443));
#7555=DIRECTION('',(0.866025403784443,0.,0.499999999999992));
#7556=DIRECTION('center_axis',(-0.866025403784443,0.,-0.499999999999992));
#7557=DIRECTION('ref_axis',(-0.499999999999992,0.,0.866025403784443));
#7558=DIRECTION('',(0.866025403784443,0.,0.499999999999993));
#7559=DIRECTION('center_axis',(-0.866025403784443,0.,-0.499999999999992));
#7560=DIRECTION('ref_axis',(-0.499999999999992,0.,0.866025403784443));
#7561=DIRECTION('center_axis',(-0.866025403784443,0.,-0.499999999999992));
#7562=DIRECTION('ref_axis',(-0.499999999999992,0.,0.866025403784443));
#7563=DIRECTION('',(-0.171010071662818,-0.939692620785907,0.296198132726037));
#7564=DIRECTION('',(-0.469846310392953,0.34202014332566,0.813797681349378));
#7565=DIRECTION('',(0.171010071662822,0.93969262078591,-0.296198132726026));
#7566=DIRECTION('',(-0.321393804843259,0.766044443118992,0.556670399226406));
#7567=DIRECTION('',(0.383022221559474,0.642787609686542,-0.663413948168944));
#7568=DIRECTION('',(0.32139380484327,-0.766044443118983,-0.556670399226412));
#7569=DIRECTION('',(0.492403876506091,0.173648177666908,-0.852868531952455));
#7570=DIRECTION('',(0.0868240888334702,-0.984807753012207,-0.150383733180441));
#7571=DIRECTION('',(-0.492403876506098,-0.173648177666911,0.852868531952451));
#7572=DIRECTION('center_axis',(-0.866025403784443,0.,-0.499999999999992));
#7573=DIRECTION('ref_axis',(-0.499999999999992,0.,0.866025403784443));
#7574=DIRECTION('center_axis',(-0.866025403784436,0.,0.500000000000004));
#7575=DIRECTION('ref_axis',(-0.321393804843269,0.766044443118983,-0.556670399226412));
#7576=DIRECTION('',(-0.866025403784437,0.,0.500000000000003));
#7577=DIRECTION('center_axis',(0.866025403784436,0.,-0.500000000000004));
#7578=DIRECTION('ref_axis',(-0.500000000000004,0.,-0.866025403784436));
#7579=DIRECTION('',(-0.866025403784436,0.,0.500000000000004));
#7580=DIRECTION('center_axis',(0.866025403784436,0.,-0.500000000000004));
#7581=DIRECTION('ref_axis',(-0.500000000000004,0.,-0.866025403784436));
#7582=DIRECTION('center_axis',(-0.866025403784436,0.,0.500000000000004));
#7583=DIRECTION('ref_axis',(0.500000000000004,0.,0.866025403784436));
#7584=DIRECTION('',(-0.866025403784436,0.,0.500000000000005));
#7585=DIRECTION('center_axis',(0.866025403784436,0.,-0.500000000000004));
#7586=DIRECTION('ref_axis',(-0.500000000000004,0.,-0.866025403784436));
#7587=DIRECTION('',(-0.866025403784435,0.,0.500000000000006));
#7588=DIRECTION('center_axis',(0.866025403784436,0.,-0.500000000000004));
#7589=DIRECTION('ref_axis',(-0.500000000000004,0.,-0.866025403784436));
#7590=DIRECTION('center_axis',(-0.866025403784436,0.,0.500000000000004));
#7591=DIRECTION('ref_axis',(0.500000000000004,0.,0.866025403784436));
#7592=DIRECTION('',(-0.866025403784436,0.,0.500000000000004));
#7593=DIRECTION('center_axis',(0.866025403784436,0.,-0.500000000000004));
#7594=DIRECTION('ref_axis',(-0.500000000000004,0.,-0.866025403784436));
#7595=DIRECTION('',(-0.866025403784436,0.,0.500000000000005));
#7596=DIRECTION('center_axis',(0.866025403784436,0.,-0.500000000000004));
#7597=DIRECTION('ref_axis',(-0.500000000000004,0.,-0.866025403784436));
#7598=DIRECTION('center_axis',(0.866025403784436,0.,-0.500000000000004));
#7599=DIRECTION('ref_axis',(-0.500000000000004,0.,-0.866025403784436));
#7600=DIRECTION('',(-0.171010071662835,-0.939692620785907,-0.296198132726028));
#7601=DIRECTION('',(-0.469846310392953,0.34202014332566,-0.813797681349378));
#7602=DIRECTION('',(0.171010071662839,0.93969262078591,0.296198132726018));
#7603=DIRECTION('',(-0.321393804843267,0.766044443118985,-0.556670399226411));
#7604=DIRECTION('',(0.383022221559487,0.642787609686547,0.663413948168932));
#7605=DIRECTION('',(0.321393804843261,-0.766044443118982,0.556670399226419));
#7606=DIRECTION('',(0.492403876506108,0.173648177666911,0.852868531952445));
#7607=DIRECTION('',(0.0868240888334687,-0.984807753012208,0.150383733180434));
#7608=DIRECTION('',(-0.492403876506111,-0.173648177666932,-0.852868531952439));
#7609=DIRECTION('center_axis',(0.866025403784436,0.,-0.500000000000004));
#7610=DIRECTION('ref_axis',(-0.500000000000004,0.,-0.866025403784436));
#7611=DIRECTION('center_axis',(0.,0.,-1.));
#7612=DIRECTION('ref_axis',(-1.,0.,0.));
#7613=DIRECTION('',(0.,0.,-1.));
#7614=DIRECTION('center_axis',(0.,0.,1.));
#7615=DIRECTION('ref_axis',(1.,0.,0.));
#7616=DIRECTION('',(0.,0.,-1.));
#7617=DIRECTION('center_axis',(0.,0.,1.));
#7618=DIRECTION('ref_axis',(1.,0.,0.));
#7619=DIRECTION('center_axis',(0.,0.,-1.));
#7620=DIRECTION('ref_axis',(-1.,0.,0.));
#7621=DIRECTION('',(0.,0.,-1.));
#7622=DIRECTION('center_axis',(0.,0.,1.));
#7623=DIRECTION('ref_axis',(1.,0.,0.));
#7624=DIRECTION('',(0.,0.,-1.));
#7625=DIRECTION('center_axis',(0.,0.,1.));
#7626=DIRECTION('ref_axis',(1.,0.,0.));
#7627=DIRECTION('center_axis',(0.,0.,-1.));
#7628=DIRECTION('ref_axis',(0.642787609686533,0.766044443118984,0.));
#7629=DIRECTION('',(0.,0.,-1.));
#7630=DIRECTION('center_axis',(0.,0.,1.));
#7631=DIRECTION('ref_axis',(1.,0.,0.));
#7632=DIRECTION('',(0.,0.,-1.));
#7633=DIRECTION('center_axis',(0.,0.,1.));
#7634=DIRECTION('ref_axis',(1.,0.,0.));
#7635=DIRECTION('center_axis',(0.,0.,1.));
#7636=DIRECTION('ref_axis',(1.,0.,0.));
#7637=DIRECTION('',(0.642787609686527,0.766044443118988,0.));
#7638=DIRECTION('',(-0.766044443118964,0.642787609686556,0.));
#7639=DIRECTION('',(-0.642787609686546,-0.766044443118973,0.));
#7640=DIRECTION('',(-0.984807753012213,0.173648177666901,0.));
#7641=DIRECTION('',(-0.173648177666935,-0.984807753012207,0.));
#7642=DIRECTION('',(0.984807753012211,-0.173648177666915,0.));
#7643=DIRECTION('',(0.342020143325671,-0.939692620785908,0.));
#7644=DIRECTION('',(0.939692620785911,0.342020143325661,0.));
#7645=DIRECTION('',(-0.342020143325671,0.939692620785908,0.));
#7646=DIRECTION('center_axis',(0.,0.,1.));
#7647=DIRECTION('ref_axis',(1.,0.,0.));
#7648=DIRECTION('center_axis',(0.,-1.,0.));
#7649=DIRECTION('ref_axis',(0.,0.,-1.));
#7650=DIRECTION('center_axis',(0.,1.,0.));
#7651=DIRECTION('ref_axis',(0.,0.,1.));
#7652=DIRECTION('',(0.,1.,0.));
#7653=DIRECTION('',(0.,1.,0.));
#7654=DIRECTION('center_axis',(0.,1.,0.));
#7655=DIRECTION('ref_axis',(0.,0.,1.));
#7656=DIRECTION('center_axis',(0.,1.,0.));
#7657=DIRECTION('ref_axis',(0.,0.,1.));
#7658=DIRECTION('center_axis',(0.,1.,0.));
#7659=DIRECTION('ref_axis',(0.,0.,1.));
#7660=DIRECTION('center_axis',(0.,1.,0.));
#7661=DIRECTION('ref_axis',(0.,0.,1.));
#7662=DIRECTION('center_axis',(0.,-1.,0.));
#7663=DIRECTION('ref_axis',(0.,0.,-1.));
#7664=DIRECTION('center_axis',(0.,1.,0.));
#7665=DIRECTION('ref_axis',(0.,0.,1.));
#7666=DIRECTION('center_axis',(0.,1.,0.));
#7667=DIRECTION('ref_axis',(0.,0.,1.));
#7668=DIRECTION('',(0.,1.,0.));
#7669=DIRECTION('center_axis',(0.,1.,0.));
#7670=DIRECTION('ref_axis',(0.,0.,1.));
#7671=DIRECTION('center_axis',(0.,0.,1.));
#7672=DIRECTION('ref_axis',(1.,0.,0.));
#7673=DIRECTION('center_axis',(0.,0.,1.));
#7674=DIRECTION('ref_axis',(1.,0.,0.));
#7675=DIRECTION('',(0.,0.,-1.));
#7676=DIRECTION('center_axis',(0.,0.,1.));
#7677=DIRECTION('ref_axis',(1.,0.,0.));
#7678=DIRECTION('center_axis',(0.,0.,1.));
#7679=DIRECTION('ref_axis',(1.,0.,0.));
#7680=DIRECTION('',(-0.642787609686536,-0.766044443118981,0.));
#7681=DIRECTION('',(-0.76604444311897,0.642787609686548,0.));
#7682=DIRECTION('',(-0.642787609686528,-0.766044443118987,0.));
#7683=DIRECTION('',(-0.342020143325666,0.939692620785909,0.));
#7684=DIRECTION('',(0.939692620785913,0.342020143325658,0.));
#7685=DIRECTION('',(-0.342020143325671,0.939692620785908,0.));
#7686=DIRECTION('',(0.984807753012212,-0.173648177666909,0.));
#7687=DIRECTION('',(-0.173648177666936,-0.984807753012207,0.));
#7688=DIRECTION('',(0.98480775301221,-0.173648177666918,0.));
#7689=DIRECTION('center_axis',(0.,0.,-1.));
#7690=DIRECTION('ref_axis',(-1.,0.,0.));
#7691=DIRECTION('center_axis',(0.,0.,1.));
#7692=DIRECTION('ref_axis',(1.,0.,0.));
#7693=DIRECTION('center_axis',(0.,0.,1.));
#7694=DIRECTION('ref_axis',(1.,0.,0.));
#7695=DIRECTION('',(0.,0.,1.));
#7696=DIRECTION('center_axis',(0.,0.,1.));
#7697=DIRECTION('ref_axis',(1.,0.,0.));
#7698=DIRECTION('',(0.,0.,1.));
#7699=DIRECTION('center_axis',(0.,0.,1.));
#7700=DIRECTION('ref_axis',(1.,0.,0.));
#7701=DIRECTION('',(0.707106781186548,8.65956056235493E-17,-0.707106781186548));
#7702=DIRECTION('center_axis',(0.866025403784443,0.,-0.499999999999992));
#7703=DIRECTION('ref_axis',(-0.499999999999992,0.,-0.866025403784443));
#7704=DIRECTION('center_axis',(0.866025403784443,0.,-0.499999999999992));
#7705=DIRECTION('ref_axis',(-0.499999999999992,0.,-0.866025403784443));
#7706=DIRECTION('',(-0.866025403784443,0.,0.499999999999992));
#7707=DIRECTION('center_axis',(-0.866025403784436,0.,-0.500000000000004));
#7708=DIRECTION('ref_axis',(-0.500000000000004,0.,0.866025403784436));
#7709=DIRECTION('center_axis',(-0.866025403784436,0.,-0.500000000000004));
#7710=DIRECTION('ref_axis',(-0.500000000000004,0.,0.866025403784436));
#7711=DIRECTION('',(0.866025403784436,0.,0.500000000000004));
#7712=DIRECTION('center_axis',(-0.866025403784443,0.,-0.499999999999992));
#7713=DIRECTION('ref_axis',(-0.499999999999992,0.,0.866025403784443));
#7714=DIRECTION('center_axis',(-0.866025403784443,0.,-0.499999999999992));
#7715=DIRECTION('ref_axis',(-0.499999999999992,0.,0.866025403784443));
#7716=DIRECTION('',(0.171010071662833,0.939692620785909,-0.296198132726024));
#7717=DIRECTION('',(-0.492403876506096,-0.17364817766691,0.852868531952452));
#7718=DIRECTION('',(0.0868240888334701,-0.984807753012206,-0.150383733180445));
#7719=DIRECTION('',(-0.4924038765061,-0.173648177666906,0.85286853195245));
#7720=DIRECTION('',(0.321393804843263,-0.766044443118983,-0.556670399226417));
#7721=DIRECTION('',(0.383022221559485,0.642787609686548,-0.663413948168932));
#7722=DIRECTION('',(0.321393804843258,-0.766044443118986,-0.556670399226415));
#7723=DIRECTION('',(0.171010071662833,0.939692620785909,-0.296198132726024));
#7724=DIRECTION('',(-0.469846310392945,0.342020143325657,0.813797681349384));
#7725=DIRECTION('center_axis',(0.866025403784443,0.,0.499999999999992));
#7726=DIRECTION('ref_axis',(0.499999999999992,0.,-0.866025403784443));
#7727=DIRECTION('center_axis',(-0.866025403784445,0.,-0.49999999999999));
#7728=DIRECTION('ref_axis',(-0.49999999999999,0.,0.866025403784445));
#7729=DIRECTION('center_axis',(-0.866025403784445,0.,-0.49999999999999));
#7730=DIRECTION('ref_axis',(-0.49999999999999,0.,0.866025403784445));
#7731=DIRECTION('',(-0.866025403784443,0.,-0.499999999999992));
#7732=DIRECTION('center_axis',(0.866025403784436,0.,-0.500000000000004));
#7733=DIRECTION('ref_axis',(-0.500000000000004,0.,-0.866025403784436));
#7734=DIRECTION('center_axis',(0.866025403784436,0.,-0.500000000000004));
#7735=DIRECTION('ref_axis',(-0.500000000000004,0.,-0.866025403784436));
#7736=DIRECTION('',(0.171010071662833,0.939692620785909,0.296198132726024));
#7737=DIRECTION('',(-0.49240387650611,-0.173648177666926,-0.852868531952441));
#7738=DIRECTION('',(0.0868240888334687,-0.984807753012208,0.150383733180434));
#7739=DIRECTION('',(-0.492403876506114,-0.173648177666907,-0.852868531952442));
#7740=DIRECTION('',(0.321393804843267,-0.766044443118988,0.556670399226408));
#7741=DIRECTION('',(0.383022221559495,0.64278760968655,0.663413948168925));
#7742=DIRECTION('',(0.321393804843269,-0.766044443118987,0.556670399226408));
#7743=DIRECTION('',(0.171010071662833,0.939692620785909,0.296198132726024));
#7744=DIRECTION('',(-0.469846310392969,0.342020143325655,-0.813797681349371));
#7745=DIRECTION('center_axis',(-0.866025403784436,0.,0.500000000000004));
#7746=DIRECTION('ref_axis',(0.500000000000004,0.,0.866025403784436));
#7747=DIRECTION('center_axis',(0.866025403784436,0.,-0.500000000000004));
#7748=DIRECTION('ref_axis',(-0.500000000000004,0.,-0.866025403784436));
#7749=DIRECTION('center_axis',(0.866025403784436,0.,-0.500000000000004));
#7750=DIRECTION('ref_axis',(-0.500000000000004,0.,-0.866025403784436));
#7751=DIRECTION('',(0.866025403784436,0.,-0.500000000000004));
#7752=DIRECTION('center_axis',(-0.866025403784436,0.,-0.500000000000004));
#7753=DIRECTION('ref_axis',(-0.500000000000004,0.,0.866025403784436));
#7754=DIRECTION('',(-0.866025403784436,0.,-0.500000000000004));
#7755=DIRECTION('center_axis',(0.866025403784443,0.,-0.499999999999992));
#7756=DIRECTION('ref_axis',(-0.499999999999992,0.,-0.866025403784443));
#7757=DIRECTION('',(0.866025403784443,0.,-0.499999999999992));
#7758=DIRECTION('center_axis',(0.866025403784436,0.,-0.500000000000004));
#7759=DIRECTION('ref_axis',(-0.500000000000004,0.,-0.866025403784436));
#7760=DIRECTION('',(-0.965925826289069,8.65956056235496E-17,-0.258819045102519));
#7761=DIRECTION('center_axis',(-0.866025403784445,0.,-0.49999999999999));
#7762=DIRECTION('ref_axis',(-0.49999999999999,0.,0.866025403784445));
#7763=DIRECTION('',(0.258819045102533,8.65956056235492E-17,0.965925826289065));
#7764=DIRECTION('center_axis',(0.,1.,0.));
#7765=DIRECTION('ref_axis',(0.,0.,1.));
#7766=DIRECTION('center_axis',(0.,1.,0.));
#7767=DIRECTION('ref_axis',(0.,0.,1.));
#7768=DIRECTION('center_axis',(0.,-1.,0.));
#7769=DIRECTION('ref_axis',(0.,0.,-1.));
#7770=DIRECTION('',(0.,-1.,0.));
#7771=DIRECTION('',(0.,-1.,0.));
#7772=DIRECTION('center_axis',(-0.939692620785908,-0.342020143325669,0.));
#7773=DIRECTION('ref_axis',(0.,0.,1.));
#7774=DIRECTION('',(0.,0.,1.));
#7775=DIRECTION('center_axis',(0.939692620785908,0.342020143325669,0.));
#7776=DIRECTION('ref_axis',(0.,0.,-1.));
#7777=DIRECTION('',(0.,0.,-1.));
#7778=DIRECTION('center_axis',(0.342020143325655,-0.939692620785914,0.));
#7779=DIRECTION('ref_axis',(0.,0.,-1.));
#7780=DIRECTION('center_axis',(0.173648177666921,0.98480775301221,0.));
#7781=DIRECTION('ref_axis',(0.,0.,1.));
#7782=DIRECTION('',(0.,0.,1.));
#7783=DIRECTION('center_axis',(-0.173648177666921,-0.98480775301221,0.));
#7784=DIRECTION('ref_axis',(0.,0.,-1.));
#7785=DIRECTION('',(0.,0.,-1.));
#7786=DIRECTION('center_axis',(-0.984807753012207,0.173648177666936,0.));
#7787=DIRECTION('ref_axis',(0.,0.,1.));
#7788=DIRECTION('center_axis',(0.766044443118981,-0.642787609686535,0.));
#7789=DIRECTION('ref_axis',(0.,0.,-1.));
#7790=DIRECTION('',(0.,0.,1.));
#7791=DIRECTION('center_axis',(-0.766044443118981,0.642787609686535,0.));
#7792=DIRECTION('ref_axis',(0.,0.,1.));
#7793=DIRECTION('',(0.,0.,-1.));
#7794=DIRECTION('center_axis',(0.642787609686547,0.766044443118972,0.));
#7795=DIRECTION('ref_axis',(0.,0.,-1.));
#7796=DIRECTION('center_axis',(-0.0868240888334609,0.98480775301221,-0.150383733180426));
#7797=DIRECTION('ref_axis',(0.,0.150953786239872,0.98854082081614));
#7798=DIRECTION('',(0.866025403784436,0.,-0.500000000000005));
#7799=DIRECTION('center_axis',(0.0868240888334609,-0.98480775301221,0.150383733180426));
#7800=DIRECTION('ref_axis',(0.,-0.150953786239872,-0.98854082081614));
#7801=DIRECTION('',(-0.866025403784436,0.,0.500000000000005));
#7802=DIRECTION('center_axis',(0.492403876506108,0.173648177666936,0.85286853195244));
#7803=DIRECTION('ref_axis',(0.866025403784436,0.,-0.500000000000004));
#7804=DIRECTION('center_axis',(-0.383022221559494,-0.642787609686535,-0.66341394816894));
#7805=DIRECTION('ref_axis',(-0.866025403784436,0.,0.500000000000004));
#7806=DIRECTION('',(0.866025403784436,0.,-0.500000000000005));
#7807=DIRECTION('center_axis',(0.383022221559494,0.642787609686535,0.66341394816894));
#7808=DIRECTION('ref_axis',(0.866025403784436,0.,-0.500000000000004));
#7809=DIRECTION('',(-0.866025403784436,0.,0.500000000000005));
#7810=DIRECTION('center_axis',(-0.321393804843276,0.766044443118972,-0.556670399226425));
#7811=DIRECTION('ref_axis',(-0.866025403784436,0.,0.500000000000004));
#7812=DIRECTION('center_axis',(0.469846310392958,-0.342020143325669,0.813797681349371));
#7813=DIRECTION('ref_axis',(0.866025403784436,0.,-0.500000000000004));
#7814=DIRECTION('',(0.866025403784437,0.,-0.500000000000003));
#7815=DIRECTION('center_axis',(-0.469846310392958,0.342020143325669,-0.813797681349371));
#7816=DIRECTION('ref_axis',(-0.866025403784436,0.,0.500000000000004));
#7817=DIRECTION('',(-0.866025403784437,0.,0.500000000000003));
#7818=DIRECTION('center_axis',(-0.171010071662829,-0.939692620785914,-0.296198132726011));
#7819=DIRECTION('ref_axis',(0.,0.300626578483209,-0.953741925422952));
#7820=DIRECTION('center_axis',(-0.0868240888334589,0.98480775301221,0.150383733180428));
#7821=DIRECTION('ref_axis',(0.,-0.150953786239873,0.988540820816139));
#7822=DIRECTION('',(-0.866025403784443,0.,-0.499999999999992));
#7823=DIRECTION('center_axis',(0.0868240888334589,-0.98480775301221,-0.150383733180428));
#7824=DIRECTION('ref_axis',(0.,0.150953786239873,-0.988540820816139));
#7825=DIRECTION('',(0.866025403784443,0.,0.499999999999992));
#7826=DIRECTION('center_axis',(0.492403876506096,0.173648177666936,-0.852868531952447));
#7827=DIRECTION('ref_axis',(-0.866025403784443,0.,-0.499999999999992));
#7828=DIRECTION('center_axis',(-0.383022221559485,-0.642787609686535,0.663413948168945));
#7829=DIRECTION('ref_axis',(0.866025403784443,0.,0.499999999999992));
#7830=DIRECTION('',(-0.866025403784443,0.,-0.499999999999992));
#7831=DIRECTION('center_axis',(0.383022221559485,0.642787609686535,-0.663413948168945));
#7832=DIRECTION('ref_axis',(-0.866025403784443,0.,-0.499999999999992));
#7833=DIRECTION('',(0.866025403784443,0.,0.499999999999992));
#7834=DIRECTION('center_axis',(-0.321393804843268,0.766044443118972,0.556670399226429));
#7835=DIRECTION('ref_axis',(0.866025403784443,0.,0.499999999999992));
#7836=DIRECTION('center_axis',(0.469846310392947,-0.342020143325669,-0.813797681349378));
#7837=DIRECTION('ref_axis',(-0.866025403784443,0.,-0.499999999999992));
#7838=DIRECTION('',(-0.866025403784443,0.,-0.499999999999992));
#7839=DIRECTION('center_axis',(-0.469846310392947,0.342020143325669,0.813797681349378));
#7840=DIRECTION('ref_axis',(0.866025403784443,0.,0.499999999999992));
#7841=DIRECTION('',(0.866025403784443,0.,0.499999999999992));
#7842=DIRECTION('center_axis',(-0.171010071662825,-0.939692620785914,0.296198132726013));
#7843=DIRECTION('ref_axis',(0.,-0.300626578483211,-0.953741925422951));
#11498=CARTESIAN_POINT('',(0.,0.,0.));
#11499=CARTESIAN_POINT('Origin',(3.21444260098502E-12,109.,121.5));
#11500=CARTESIAN_POINT('',(-11.2583302491955,102.499999999999,121.5));
#11501=CARTESIAN_POINT('',(11.2583302492019,115.500000000001,121.5));
#11502=CARTESIAN_POINT('Origin',(3.21444260098502E-12,109.,121.5));
#11503=CARTESIAN_POINT('',(9.52627944163062,114.499999999999,121.5));
#11504=CARTESIAN_POINT('',(11.2583302492019,115.500000000001,121.5));
#11505=CARTESIAN_POINT('',(-9.52627944162417,103.500000000001,121.5));
#11506=CARTESIAN_POINT('Origin',(3.21444260098502E-12,109.,121.5));
#11507=CARTESIAN_POINT('',(-9.52627944162417,103.500000000001,121.5));
#11508=CARTESIAN_POINT('Origin',(11.2583302492011,115.500000000001,60.4999999999998));
#11509=CARTESIAN_POINT('',(9.52627944162984,114.499999999999,65.5));
#11510=CARTESIAN_POINT('',(11.2583302491965,115.499999999998,65.5));
#11511=CARTESIAN_POINT('',(9.52627944162984,114.499999999999,65.5));
#11512=CARTESIAN_POINT('',(9.52627944162984,114.499999999999,65.5));
#11513=CARTESIAN_POINT('',(11.2583302492012,115.500000000001,65.5));
#11514=CARTESIAN_POINT('Origin',(2.36789754470834E-12,109.,60.5));
#11515=CARTESIAN_POINT('',(-9.52627944162487,103.500000000001,65.5));
#11516=CARTESIAN_POINT('Origin',(2.43784159525973E-12,109.,65.5));
#11517=CARTESIAN_POINT('',(-9.52627944162496,103.500000000001,65.5));
#11518=CARTESIAN_POINT('Origin',(-9.52627944162501,103.500000000001,60.5000000000001));
#11519=CARTESIAN_POINT('',(-11.2583302491953,102.5,65.5));
#11520=CARTESIAN_POINT('',(-11.2583302491953,102.5,65.5));
#11521=CARTESIAN_POINT('',(-11.2583302491962,102.499999999999,65.5));
#11522=CARTESIAN_POINT('Origin',(2.36789754470834E-12,109.,60.5));
#11523=CARTESIAN_POINT('Origin',(4.79810263127257E-15,109.,65.5));
#11524=CARTESIAN_POINT('Origin',(4.79810263127257E-15,109.,65.5));
#11525=CARTESIAN_POINT('Origin',(-115.614391405224,109.,-78.7499999999976));
#11526=CARTESIAN_POINT('',(-109.985226280625,102.499999999999,-88.4999999999985));
#11527=CARTESIAN_POINT('',(-121.243556529823,115.500000000001,-68.9999999999967));
#11528=CARTESIAN_POINT('Origin',(-115.614391405224,109.,-78.7499999999976));
#11529=CARTESIAN_POINT('',(-120.377531126037,114.499999999999,-70.4999999999988));
#11530=CARTESIAN_POINT('',(-121.243556529823,115.500000000001,-68.9999999999967));
#11531=CARTESIAN_POINT('',(-110.85125168441,103.500000000001,-86.9999999999964));
#11532=CARTESIAN_POINT('Origin',(-115.614391405224,109.,-78.7499999999976));
#11533=CARTESIAN_POINT('',(-110.85125168441,103.500000000001,-86.9999999999964));
#11534=CARTESIAN_POINT('Origin',(-68.416006898972,115.500000000001,-38.4999999999972));
#11535=CARTESIAN_POINT('',(-71.8801085141086,114.499999999999,-42.4999999999993));
#11536=CARTESIAN_POINT('',(-72.7461339178932,115.499999999999,-40.9999999999989));
#11537=CARTESIAN_POINT('',(-71.8801085141086,114.499999999999,-42.4999999999993));
#11538=CARTESIAN_POINT('',(-71.8801085141086,114.499999999999,-42.4999999999993));
#11539=CARTESIAN_POINT('',(-72.7461339178942,115.500000000001,-40.9999999999972));
#11540=CARTESIAN_POINT('Origin',(-62.7868417743727,109.,-48.2499999999981));
#11541=CARTESIAN_POINT('',(-62.3538290724813,103.500000000001,-58.9999999999969));
#11542=CARTESIAN_POINT('Origin',(-67.116968793295,109.,-50.7499999999981));
#11543=CARTESIAN_POINT('',(-62.3538290724813,103.500000000001,-58.9999999999969));
#11544=CARTESIAN_POINT('Origin',(-58.0237020535591,103.500000000001,-56.4999999999969));
#11545=CARTESIAN_POINT('',(-61.4878036686957,102.499999999999,-60.499999999999));
#11546=CARTESIAN_POINT('',(-61.4878036686957,102.499999999999,-60.499999999999));
#11547=CARTESIAN_POINT('',(-61.4878036686957,102.499999999999,-60.499999999999));
#11548=CARTESIAN_POINT('Origin',(-62.7868417743727,109.,-48.2499999999981));
#11549=CARTESIAN_POINT('Origin',(-67.1169687932943,109.,-50.7499999999993));
#11550=CARTESIAN_POINT('Origin',(-67.1169687932943,109.,-50.7499999999993));
#11551=CARTESIAN_POINT('Origin',(115.614391405221,109.,-78.7500000000032));
#11552=CARTESIAN_POINT('',(121.24355652982,102.499999999999,-69.0000000000025));
#11553=CARTESIAN_POINT('',(109.985226280621,115.500000000001,-88.500000000004));
#11554=CARTESIAN_POINT('Origin',(115.614391405221,109.,-78.7500000000032));
#11555=CARTESIAN_POINT('',(110.851251684407,114.499999999999,-87.0000000000019));
#11556=CARTESIAN_POINT('',(109.985226280621,115.500000000001,-88.500000000004));
#11557=CARTESIAN_POINT('',(120.377531126034,103.500000000001,-70.5000000000045));
#11558=CARTESIAN_POINT('Origin',(115.614391405221,109.,-78.7500000000032));
#11559=CARTESIAN_POINT('',(120.377531126034,103.500000000001,-70.5000000000045));
#11560=CARTESIAN_POINT('Origin',(57.1576766497708,115.500000000001,-58.000000000003));
#11561=CARTESIAN_POINT('',(62.3538290724788,114.499999999999,-59.0000000000011));
#11562=CARTESIAN_POINT('',(61.4878036686952,115.499999999998,-60.4999999999996));
#11563=CARTESIAN_POINT('',(62.3538290724788,114.499999999999,-59.0000000000011));
#11564=CARTESIAN_POINT('',(62.3538290724788,114.499999999999,-59.0000000000011));
#11565=CARTESIAN_POINT('',(61.4878036686932,115.500000000001,-60.5000000000032));
#11566=CARTESIAN_POINT('Origin',(62.7868417743704,109.,-48.2500000000022));
#11567=CARTESIAN_POINT('',(71.8801085141063,103.500000000001,-42.5000000000036));
#11568=CARTESIAN_POINT('Origin',(67.1169687932926,109.,-50.7500000000023));
#11569=CARTESIAN_POINT('',(71.8801085141063,103.500000000001,-42.5000000000036));
#11570=CARTESIAN_POINT('Origin',(67.5499814951842,103.500000000001,-40.0000000000036));
#11571=CARTESIAN_POINT('',(72.7461339178917,102.5,-41.0000000000018));
#11572=CARTESIAN_POINT('',(72.7461339178918,102.5,-41.0000000000018));
#11573=CARTESIAN_POINT('',(72.7461339178919,102.499999999999,-41.0000000000015));
#11574=CARTESIAN_POINT('Origin',(62.7868417743704,109.,-48.2500000000022));
#11575=CARTESIAN_POINT('Origin',(67.1169687932938,109.,-50.7500000000002));
#11576=CARTESIAN_POINT('Origin',(67.1169687932938,109.,-50.7500000000002));
#11577=CARTESIAN_POINT('Origin',(-67.1169687932943,109.,-50.7499999999992));
#11578=CARTESIAN_POINT('',(-64.7881663535555,123.258566435188,-54.7836041464173));
#11579=CARTESIAN_POINT('',(-61.3240647384177,123.258566435188,-52.7836041464173));
#11580=CARTESIAN_POINT('',(-64.7881663535555,123.258566435188,-54.7836041464173));
#11581=CARTESIAN_POINT('',(-74.5423344792075,106.889128681836,-37.8888893672188));
#11582=CARTESIAN_POINT('Origin',(-67.1169687932943,109.,-50.7499999999992));
#11583=CARTESIAN_POINT('',(-71.0782328640697,106.889128681836,-35.8888893672189));
#11584=CARTESIAN_POINT('',(-74.5423344792075,106.889128681836,-37.8888893672188));
#11585=CARTESIAN_POINT('Origin',(-63.6528671781565,109.,-48.7499999999993));
#11586=CARTESIAN_POINT('Origin',(-67.1169687932943,109.,-50.7499999999992));
#11587=CARTESIAN_POINT('',(-60.8542184280248,122.916546291862,-53.5974018277667));
#11588=CARTESIAN_POINT('',(-64.3183200431626,122.916546291862,-55.5974018277666));
#11589=CARTESIAN_POINT('',(-64.3183200431626,122.916546291862,-55.5974018277666));
#11590=CARTESIAN_POINT('',(-58.6431280208156,97.837112635988,-57.4271227531812));
#11591=CARTESIAN_POINT('Origin',(-63.6528671781565,109.,-48.7499999999993));
#11592=CARTESIAN_POINT('',(-62.1072296359534,97.837112635988,-59.4271227531812));
#11593=CARTESIAN_POINT('',(-62.1072296359534,97.837112635988,-59.4271227531812));
#11594=CARTESIAN_POINT('Origin',(-67.1169687932943,109.,-50.7499999999992));
#11595=CARTESIAN_POINT('Origin',(-67.1169687932943,109.,-50.7499999999992));
#11596=CARTESIAN_POINT('',(-59.0261502423751,97.1943250263015,-56.7637088050123));
#11597=CARTESIAN_POINT('',(-62.4902518575129,97.1943250263015,-58.7637088050122));
#11598=CARTESIAN_POINT('',(-62.4902518575129,97.1943250263015,-58.7637088050122));
#11599=CARTESIAN_POINT('',(-70.9914087752362,105.904320928824,-36.0392731003993));
#11600=CARTESIAN_POINT('Origin',(-63.6528671781565,109.,-48.7499999999993));
#11601=CARTESIAN_POINT('',(-74.455510390374,105.904320928824,-38.0392731003992));
#11602=CARTESIAN_POINT('',(-74.455510390374,105.904320928824,-38.0392731003992));
#11603=CARTESIAN_POINT('Origin',(-67.1169687932943,109.,-50.7499999999992));
#11604=CARTESIAN_POINT('Origin',(-67.1169687932943,109.,-50.7499999999992));
#11605=CARTESIAN_POINT('',(-64.9661511107924,122.280548232157,-54.4753255039102));
#11606=CARTESIAN_POINT('',(-64.7881663535555,123.258566435188,-54.7836041464173));
#11607=CARTESIAN_POINT('',(-64.4963048003994,121.938528088831,-55.2891231852596));
#11608=CARTESIAN_POINT('',(-64.4963048003994,121.938528088831,-55.2891231852596));
#11609=CARTESIAN_POINT('',(-64.4963048003994,121.938528088831,-55.2891231852596));
#11610=CARTESIAN_POINT('',(-62.4417315619291,98.6344003800105,-58.8477484221616));
#11611=CARTESIAN_POINT('',(-62.1072296359534,97.837112635988,-59.4271227531812));
#11612=CARTESIAN_POINT('',(-62.8247537834885,97.9916127703239,-58.1843344739927));
#11613=CARTESIAN_POINT('',(-62.8247537834885,97.9916127703239,-58.1843344739927));
#11614=CARTESIAN_POINT('',(-62.8247537834886,97.9916127703239,-58.1843344739927));
#11615=CARTESIAN_POINT('',(-73.9430237071614,106.085051387833,-38.9269260739259));
#11616=CARTESIAN_POINT('',(-74.455510390374,105.904320928824,-38.0392731003992));
#11617=CARTESIAN_POINT('',(-74.0298477959949,107.069859140845,-38.7765423407454));
#11618=CARTESIAN_POINT('',(-74.0298477959949,107.069859140845,-38.7765423407454));
#11619=CARTESIAN_POINT('',(-74.0298477959949,107.069859140845,-38.7765423407454));
#11620=CARTESIAN_POINT('',(-60.6169687932938,109.,-62.0083302491979));
#11621=CARTESIAN_POINT('Origin',(-67.1169687932943,109.,-50.7499999999993));
#11622=CARTESIAN_POINT('Origin',(67.1169687932938,109.,-50.7500000000002));
#11623=CARTESIAN_POINT('',(69.4457712330326,123.258566435188,-46.7163958535822));
#11624=CARTESIAN_POINT('',(65.9816696178948,123.258566435188,-44.7163958535822));
#11625=CARTESIAN_POINT('',(69.4457712330326,123.258566435188,-46.7163958535822));
#11626=CARTESIAN_POINT('',(59.6916031073804,106.889128681836,-63.6111106327805));
#11627=CARTESIAN_POINT('Origin',(67.1169687932938,109.,-50.7500000000002));
#11628=CARTESIAN_POINT('',(56.2275014922427,106.889128681836,-61.6111106327805));
#11629=CARTESIAN_POINT('',(59.6916031073804,106.889128681836,-63.6111106327805));
#11630=CARTESIAN_POINT('Origin',(63.652867178156,109.,-48.7500000000002));
#11631=CARTESIAN_POINT('Origin',(67.1169687932938,109.,-50.7500000000002));
#11632=CARTESIAN_POINT('',(66.4515159282878,122.916546291862,-43.9025981722328));
#11633=CARTESIAN_POINT('',(69.9156175434256,122.916546291862,-45.9025981722328));
#11634=CARTESIAN_POINT('',(69.9156175434256,122.916546291862,-45.9025981722328));
#11635=CARTESIAN_POINT('',(68.662606335497,97.837112635988,-40.0728772468183));
#11636=CARTESIAN_POINT('Origin',(63.652867178156,109.,-48.7500000000002));
#11637=CARTESIAN_POINT('',(72.1267079506348,97.837112635988,-42.0728772468184));
#11638=CARTESIAN_POINT('',(72.1267079506348,97.837112635988,-42.0728772468184));
#11639=CARTESIAN_POINT('Origin',(67.1169687932938,109.,-50.7500000000002));
#11640=CARTESIAN_POINT('Origin',(67.1169687932938,109.,-50.7500000000002));
#11641=CARTESIAN_POINT('',(68.2795841139375,97.1943250263015,-40.7362911949873));
#11642=CARTESIAN_POINT('',(71.7436857290753,97.1943250263015,-42.7362911949873));
#11643=CARTESIAN_POINT('',(71.7436857290753,97.1943250263015,-42.7362911949873));
#11644=CARTESIAN_POINT('',(56.3143255810761,105.904320928824,-61.4607268996001));
#11645=CARTESIAN_POINT('Origin',(63.652867178156,109.,-48.7500000000002));
#11646=CARTESIAN_POINT('',(59.7784271962139,105.904320928824,-63.4607268996001));
#11647=CARTESIAN_POINT('',(59.7784271962139,105.904320928824,-63.4607268996001));
#11648=CARTESIAN_POINT('Origin',(67.1169687932938,109.,-50.7500000000002));
#11649=CARTESIAN_POINT('Origin',(67.1169687932938,109.,-50.7500000000002));
#11650=CARTESIAN_POINT('',(69.2677864757957,122.280548232157,-47.0246744960893));
#11651=CARTESIAN_POINT('',(69.4457712330326,123.258566435188,-46.7163958535822));
#11652=CARTESIAN_POINT('',(69.7376327861887,121.938528088831,-46.2108768147398));
#11653=CARTESIAN_POINT('',(69.7376327861887,121.938528088831,-46.2108768147398));
#11654=CARTESIAN_POINT('',(69.7376327861887,121.938528088831,-46.2108768147399));
#11655=CARTESIAN_POINT('',(71.7922060246591,98.6344003800105,-42.6522515778379));
#11656=CARTESIAN_POINT('',(72.1267079506348,97.837112635988,-42.0728772468184));
#11657=CARTESIAN_POINT('',(71.4091838030996,97.991612770324,-43.3156655260068));
#11658=CARTESIAN_POINT('',(71.4091838030996,97.991612770324,-43.3156655260068));
#11659=CARTESIAN_POINT('',(71.4091838030996,97.9916127703239,-43.3156655260069));
#11660=CARTESIAN_POINT('',(60.2909138794264,106.085051387833,-62.5730739260735));
#11661=CARTESIAN_POINT('',(59.7784271962139,105.904320928824,-63.4607268996001));
#11662=CARTESIAN_POINT('',(60.204089790593,107.069859140845,-62.7234576592539));
#11663=CARTESIAN_POINT('',(60.204089790593,107.069859140845,-62.7234576592539));
#11664=CARTESIAN_POINT('',(60.2040897905929,107.069859140845,-62.7234576592539));
#11665=CARTESIAN_POINT('',(73.6169687932943,109.,-39.4916697508016));
#11666=CARTESIAN_POINT('Origin',(67.1169687932938,109.,-50.7500000000002));
#11667=CARTESIAN_POINT('Origin',(4.79810263127257E-15,109.,65.5));
#11668=CARTESIAN_POINT('',(-10.019478314682,97.837112635988,65.5));
#11669=CARTESIAN_POINT('',(-10.019478314682,97.837112635988,61.5));
#11670=CARTESIAN_POINT('',(-10.019478314682,97.837112635988,65.5));
#11671=CARTESIAN_POINT('',(-5.59729750026353,122.916546291862,65.5));
#11672=CARTESIAN_POINT('Origin',(4.79810263127257E-15,109.,65.5));
#11673=CARTESIAN_POINT('',(-5.59729750026353,122.916546291862,61.5));
#11674=CARTESIAN_POINT('',(-5.59729750026353,122.916546291862,65.5));
#11675=CARTESIAN_POINT('Origin',(4.79810263127257E-15,109.,61.5));
#11676=CARTESIAN_POINT('Origin',(4.79810263127257E-15,109.,65.5));
#11677=CARTESIAN_POINT('',(-9.25343387156297,97.1943250263015,61.5));
#11678=CARTESIAN_POINT('',(-9.25343387156298,97.1943250263015,65.5));
#11679=CARTESIAN_POINT('',(-9.25343387156297,97.1943250263015,65.5));
#11680=CARTESIAN_POINT('',(14.6770831941597,105.904320928824,61.5));
#11681=CARTESIAN_POINT('Origin',(4.79810263127257E-15,109.,61.5));
#11682=CARTESIAN_POINT('',(14.6770831941597,105.904320928824,65.5));
#11683=CARTESIAN_POINT('',(14.6770831941597,105.904320928824,65.5));
#11684=CARTESIAN_POINT('Origin',(4.79810263127257E-15,109.,65.5));
#11685=CARTESIAN_POINT('Origin',(4.79810263127257E-15,109.,65.5));
#11686=CARTESIAN_POINT('',(14.8507313718266,106.889128681836,61.5));
#11687=CARTESIAN_POINT('',(14.8507313718266,106.889128681836,65.5));
#11688=CARTESIAN_POINT('',(14.8507313718266,106.889128681836,65.5));
#11689=CARTESIAN_POINT('',(-4.65760487947762,123.258566435188,61.5));
#11690=CARTESIAN_POINT('Origin',(4.79810263127257E-15,109.,61.5));
#11691=CARTESIAN_POINT('',(-4.65760487947762,123.258566435188,65.5));
#11692=CARTESIAN_POINT('',(-4.65760487947762,123.258566435188,65.5));
#11693=CARTESIAN_POINT('Origin',(4.79810263127257E-15,109.,65.5));
#11694=CARTESIAN_POINT('Origin',(4.79810263127257E-15,109.,65.5));
#11695=CARTESIAN_POINT('',(-9.35047446273056,98.6344003800105,65.5));
#11696=CARTESIAN_POINT('',(-10.019478314682,97.837112635988,65.5));
#11697=CARTESIAN_POINT('',(-8.58443001961159,97.9916127703239,65.5));
#11698=CARTESIAN_POINT('',(-8.58443001961159,97.9916127703239,65.5));
#11699=CARTESIAN_POINT('',(-8.5844300196116,97.9916127703239,65.5));
#11700=CARTESIAN_POINT('',(13.6521098277345,106.085051387833,65.5));
#11701=CARTESIAN_POINT('',(14.6770831941597,105.904320928824,65.5));
#11702=CARTESIAN_POINT('',(13.8257580054015,107.069859140845,65.5));
#11703=CARTESIAN_POINT('',(13.8257580054015,107.069859140845,65.5));
#11704=CARTESIAN_POINT('',(13.8257580054015,107.069859140845,65.5));
#11705=CARTESIAN_POINT('',(-4.30163536500389,122.280548232157,65.5));
#11706=CARTESIAN_POINT('',(-4.65760487947762,123.258566435188,65.5));
#11707=CARTESIAN_POINT('',(-5.2413279857898,121.938528088831,65.5));
#11708=CARTESIAN_POINT('',(-5.2413279857898,121.938528088831,65.5));
#11709=CARTESIAN_POINT('',(-5.24132798578981,121.938528088831,65.5));
#11710=CARTESIAN_POINT('',(-13.,109.,65.5));
#11711=CARTESIAN_POINT('Origin',(4.79810263127257E-15,109.,65.5));
#11712=CARTESIAN_POINT('Origin',(0.,126.,-11.9999999999999));
#11713=CARTESIAN_POINT('',(0.,89.,16.16342581706));
#11714=CARTESIAN_POINT('Origin',(0.,89.,-11.9999999999999));
#11715=CARTESIAN_POINT('',(-1.72451246399432E-15,94.,16.16342581706));
#11716=CARTESIAN_POINT('',(-3.44902492798863E-15,126.,16.16342581706));
#11717=CARTESIAN_POINT('',(-15.,109.,11.8364962558057));
#11718=CARTESIAN_POINT('Ctrl Pts',(-15.,109.,11.8364962558057));
#11719=CARTESIAN_POINT('Ctrl Pts',(-15.,108.034202794276,11.8364962558057));
#11720=CARTESIAN_POINT('Ctrl Pts',(-14.9052762534063,107.044006310494,11.8969354528545));
#11721=CARTESIAN_POINT('Ctrl Pts',(-14.5155028930965,105.089329014181,12.1356781489979));
#11722=CARTESIAN_POINT('Ctrl Pts',(-14.2206269533151,104.124758926468,12.3135340099836));
#11723=CARTESIAN_POINT('Ctrl Pts',(-13.0649879364951,101.365664401063,12.9653152261472));
#11724=CARTESIAN_POINT('Ctrl Pts',(-11.9192829736626,99.7060795380662,13.5561572236054));
#11725=CARTESIAN_POINT('Ctrl Pts',(-9.29871093997433,97.0855075043779,14.6215293486697));
#11726=CARTESIAN_POINT('Ctrl Pts',(-7.63759490096063,95.9363382053097,15.1733726751026));
#11727=CARTESIAN_POINT('Ctrl Pts',(-4.8732166939491,94.7785446488243,15.7545840354958));
#11728=CARTESIAN_POINT('Ctrl Pts',(-3.9068153878956,94.4834357307163,15.9084529938547));
#11729=CARTESIAN_POINT('Ctrl Pts',(-1.95136354983184,94.0940942925199,16.1129353729621));
#11730=CARTESIAN_POINT('Ctrl Pts',(-0.962272640803981,94.,16.16342581706));
#11731=CARTESIAN_POINT('Ctrl Pts',(3.88578058618805E-15,94.,16.16342581706));
#11732=CARTESIAN_POINT('',(4.95933585255997E-16,124.,16.16342581706));
#11733=CARTESIAN_POINT('Ctrl Pts',(5.55111512312578E-15,124.,16.16342581706));
#11734=CARTESIAN_POINT('Ctrl Pts',(-0.962272640803984,124.,16.16342581706));
#11735=CARTESIAN_POINT('Ctrl Pts',(-1.95136354983183,123.90590570748,16.1129353729621));
#11736=CARTESIAN_POINT('Ctrl Pts',(-3.9068153878956,123.516564269284,15.9084529938547));
#11737=CARTESIAN_POINT('Ctrl Pts',(-4.87321669394909,123.221455351176,15.7545840354958));
#11738=CARTESIAN_POINT('Ctrl Pts',(-7.63759490096062,122.06366179469,15.1733726751026));
#11739=CARTESIAN_POINT('Ctrl Pts',(-9.29871093997433,120.914492495622,14.6215293486697));
#11740=CARTESIAN_POINT('Ctrl Pts',(-11.9192829736626,118.293920461934,13.5561572236054));
#11741=CARTESIAN_POINT('Ctrl Pts',(-13.0649879364951,116.634335598937,12.9653152261472));
#11742=CARTESIAN_POINT('Ctrl Pts',(-14.2206269533151,113.875241073532,12.3135340099836));
#11743=CARTESIAN_POINT('Ctrl Pts',(-14.5155028930965,112.910670985819,12.1356781489979));
#11744=CARTESIAN_POINT('Ctrl Pts',(-14.9052762534063,110.955993689506,11.8969354528545));
#11745=CARTESIAN_POINT('Ctrl Pts',(-15.,109.965797205724,11.8364962558057));
#11746=CARTESIAN_POINT('Ctrl Pts',(-15.,109.,11.8364962558057));
#11747=CARTESIAN_POINT('',(0.,126.,16.16342581706));
#11748=CARTESIAN_POINT('',(-3.44902492798863E-15,126.,16.16342581706));
#11749=CARTESIAN_POINT('Origin',(0.,126.,-11.9999999999999));
#11750=CARTESIAN_POINT('',(15.,109.,11.8364962558057));
#11751=CARTESIAN_POINT('Ctrl Pts',(15.,109.,11.8364962558057));
#11752=CARTESIAN_POINT('Ctrl Pts',(15.,109.965797205724,11.8364962558057));
#11753=CARTESIAN_POINT('Ctrl Pts',(14.9052762534063,110.955993689506,11.8969354528545));
#11754=CARTESIAN_POINT('Ctrl Pts',(14.5155028930965,112.910670985819,12.1356781489979));
#11755=CARTESIAN_POINT('Ctrl Pts',(14.2206269533151,113.875241073532,12.3135340099836));
#11756=CARTESIAN_POINT('Ctrl Pts',(13.0649879364951,116.634335598937,12.9653152261472));
#11757=CARTESIAN_POINT('Ctrl Pts',(11.9192829736626,118.293920461934,13.5561572236054));
#11758=CARTESIAN_POINT('Ctrl Pts',(9.29871093997435,120.914492495622,14.6215293486697));
#11759=CARTESIAN_POINT('Ctrl Pts',(7.63759490096064,122.06366179469,15.1733726751026));
#11760=CARTESIAN_POINT('Ctrl Pts',(4.87321669394911,123.221455351176,15.7545840354958));
#11761=CARTESIAN_POINT('Ctrl Pts',(3.90681538789561,123.516564269284,15.9084529938547));
#11762=CARTESIAN_POINT('Ctrl Pts',(1.95136354983185,123.90590570748,16.1129353729621));
#11763=CARTESIAN_POINT('Ctrl Pts',(0.962272640803995,124.,16.16342581706));
#11764=CARTESIAN_POINT('Ctrl Pts',(5.82867087928207E-15,124.,16.16342581706));
#11765=CARTESIAN_POINT('Ctrl Pts',(2.22044604925031E-15,94.,16.16342581706));
#11766=CARTESIAN_POINT('Ctrl Pts',(0.962272640803993,94.,16.16342581706));
#11767=CARTESIAN_POINT('Ctrl Pts',(1.95136354983185,94.0940942925199,16.1129353729621));
#11768=CARTESIAN_POINT('Ctrl Pts',(3.90681538789561,94.4834357307163,15.9084529938547));
#11769=CARTESIAN_POINT('Ctrl Pts',(4.87321669394911,94.7785446488243,15.7545840354958));
#11770=CARTESIAN_POINT('Ctrl Pts',(7.63759490096064,95.9363382053097,15.1733726751026));
#11771=CARTESIAN_POINT('Ctrl Pts',(9.29871093997435,97.0855075043779,14.6215293486697));
#11772=CARTESIAN_POINT('Ctrl Pts',(11.9192829736626,99.7060795380662,13.5561572236054));
#11773=CARTESIAN_POINT('Ctrl Pts',(13.0649879364951,101.365664401063,12.9653152261472));
#11774=CARTESIAN_POINT('Ctrl Pts',(14.2206269533151,104.124758926468,12.3135340099836));
#11775=CARTESIAN_POINT('Ctrl Pts',(14.5155028930965,105.089329014181,12.1356781489979));
#11776=CARTESIAN_POINT('Ctrl Pts',(14.9052762534063,107.044006310494,11.8969354528545));
#11777=CARTESIAN_POINT('Ctrl Pts',(15.,108.034202794276,11.8364962558057));
#11778=CARTESIAN_POINT('Ctrl Pts',(15.,109.,11.8364962558057));
#11779=CARTESIAN_POINT('',(-28.1430112947403,109.,-10.9278670711363));
#11780=CARTESIAN_POINT('',(-13.1430112947402,109.,-36.9086291846694));
#11781=CARTESIAN_POINT('Ctrl Pts',(-28.1430112947403,109.,-10.9278670711363));
#11782=CARTESIAN_POINT('Ctrl Pts',(-28.1430112947403,109.965797205724,-10.9278670711363));
#11783=CARTESIAN_POINT('Ctrl Pts',(-28.1479913014721,110.955993689506,-11.0401198405525));
#11784=CARTESIAN_POINT('Ctrl Pts',(-28.1598618611454,112.910670985819,-11.4970448203709));
#11785=CARTESIAN_POINT('Ctrl Pts',(-28.1664515850802,113.875241073532,-11.8413428056792));
#11786=CARTESIAN_POINT('Ctrl Pts',(-28.1530911675774,116.634335598937,-13.1680461599316));
#11787=CARTESIAN_POINT('Ctrl Pts',(-28.0919228655826,118.293920461934,-14.4556767617156));
#11788=CARTESIAN_POINT('Ctrl Pts',(-27.7042761735281,120.914492495622,-17.2578447778688));
#11789=CARTESIAN_POINT('Ctrl Pts',(-27.351628493621,122.06366179469,-18.9723351295049));
#11790=CARTESIAN_POINT('Ctrl Pts',(-26.4727831931838,123.221455351176,-21.6569625626416));
#11791=CARTESIAN_POINT('Ctrl Pts',(-26.1228369669497,123.516564269284,-22.5708251231138));
#11792=CARTESIAN_POINT('Ctrl Pts',(-25.3221979828512,123.90590570748,-24.3665372803077));
#11793=CARTESIAN_POINT('Ctrl Pts',(-24.8713785355743,124.,-25.248360356227));
#11794=CARTESIAN_POINT('Ctrl Pts',(-23.9091058947703,124.,-26.915065460833));
#11795=CARTESIAN_POINT('Ctrl Pts',(-23.3708344330193,123.90590570748,-27.7463980926544));
#11796=CARTESIAN_POINT('Ctrl Pts',(-22.2160215790541,123.516564269284,-29.3376278707409));
#11797=CARTESIAN_POINT('Ctrl Pts',(-21.5995664992347,123.221455351176,-30.0976214728542));
#11798=CARTESIAN_POINT('Ctrl Pts',(-19.7140335926603,122.06366179469,-32.2010375455977));
#11799=CARTESIAN_POINT('Ctrl Pts',(-18.4055652335537,120.914492495622,-33.3636845708009));
#11800=CARTESIAN_POINT('Ctrl Pts',(-16.17263989192,118.293920461934,-35.1004804618898));
#11801=CARTESIAN_POINT('Ctrl Pts',(-15.0881032310822,116.634335598937,-35.7972690662155));
#11802=CARTESIAN_POINT('Ctrl Pts',(-13.9458246317649,113.875241073532,-36.4721912043043));
#11803=CARTESIAN_POINT('Ctrl Pts',(-13.6443589680487,112.910670985819,-36.638633328627));
#11804=CARTESIAN_POINT('Ctrl Pts',(-13.2427150480657,110.955993689506,-36.856815612302));
#11805=CARTESIAN_POINT('Ctrl Pts',(-13.1430112947402,109.965797205724,-36.9086291846694));
#11806=CARTESIAN_POINT('Ctrl Pts',(-13.1430112947402,109.,-36.9086291846694));
#11807=CARTESIAN_POINT('Ctrl Pts',(-13.1430112947402,109.,-36.9086291846694));
#11808=CARTESIAN_POINT('Ctrl Pts',(-13.1430112947402,108.034202794276,-36.9086291846694));
#11809=CARTESIAN_POINT('Ctrl Pts',(-13.2427150480657,107.044006310494,-36.856815612302));
#11810=CARTESIAN_POINT('Ctrl Pts',(-13.6443589680487,105.089329014181,-36.638633328627));
#11811=CARTESIAN_POINT('Ctrl Pts',(-13.9458246317649,104.124758926468,-36.4721912043043));
#11812=CARTESIAN_POINT('Ctrl Pts',(-15.0881032310822,101.365664401063,-35.7972690662155));
#11813=CARTESIAN_POINT('Ctrl Pts',(-16.17263989192,99.7060795380662,-35.1004804618898));
#11814=CARTESIAN_POINT('Ctrl Pts',(-18.4055652335537,97.0855075043779,-33.3636845708009));
#11815=CARTESIAN_POINT('Ctrl Pts',(-19.7140335926603,95.9363382053097,-32.2010375455977));
#11816=CARTESIAN_POINT('Ctrl Pts',(-21.5995664992347,94.7785446488243,-30.0976214728542));
#11817=CARTESIAN_POINT('Ctrl Pts',(-22.2160215790541,94.4834357307163,-29.3376278707409));
#11818=CARTESIAN_POINT('Ctrl Pts',(-23.3708344330193,94.0940942925199,-27.7463980926544));
#11819=CARTESIAN_POINT('Ctrl Pts',(-23.9091058947703,94.,-26.915065460833));
#11820=CARTESIAN_POINT('Ctrl Pts',(-24.8713785355743,94.,-25.248360356227));
#11821=CARTESIAN_POINT('Ctrl Pts',(-25.3221979828512,94.0940942925199,-24.3665372803077));
#11822=CARTESIAN_POINT('Ctrl Pts',(-26.1228369669498,94.4834357307163,-22.5708251231138));
#11823=CARTESIAN_POINT('Ctrl Pts',(-26.4727831931838,94.7785446488243,-21.6569625626416));
#11824=CARTESIAN_POINT('Ctrl Pts',(-27.351628493621,95.9363382053097,-18.9723351295049));
#11825=CARTESIAN_POINT('Ctrl Pts',(-27.7042761735281,97.0855075043779,-17.2578447778688));
#11826=CARTESIAN_POINT('Ctrl Pts',(-28.0919228655826,99.7060795380662,-14.4556767617156));
#11827=CARTESIAN_POINT('Ctrl Pts',(-28.1530911675774,101.365664401063,-13.1680461599316));
#11828=CARTESIAN_POINT('Ctrl Pts',(-28.1664515850802,104.124758926468,-11.8413428056792));
#11829=CARTESIAN_POINT('Ctrl Pts',(-28.1598618611454,105.089329014181,-11.4970448203709));
#11830=CARTESIAN_POINT('Ctrl Pts',(-28.1479913014721,107.044006310494,-11.0401198405525));
#11831=CARTESIAN_POINT('Ctrl Pts',(-28.1430112947403,108.034202794276,-10.9278670711363));
#11832=CARTESIAN_POINT('Ctrl Pts',(-28.1430112947403,109.,-10.9278670711363));
#11833=CARTESIAN_POINT('',(13.1430112947406,109.,-36.9086291846692));
#11834=CARTESIAN_POINT('',(28.1430112947403,109.,-10.9278670711359));
#11835=CARTESIAN_POINT('Ctrl Pts',(13.1430112947406,109.,-36.9086291846692));
#11836=CARTESIAN_POINT('Ctrl Pts',(13.1430112947406,109.965797205724,-36.9086291846692));
#11837=CARTESIAN_POINT('Ctrl Pts',(13.2427150480661,110.955993689506,-36.8568156123018));
#11838=CARTESIAN_POINT('Ctrl Pts',(13.6443589680491,112.910670985819,-36.6386333286268));
#11839=CARTESIAN_POINT('Ctrl Pts',(13.9458246317653,113.875241073532,-36.4721912043041));
#11840=CARTESIAN_POINT('Ctrl Pts',(15.0881032310825,116.634335598937,-35.7972690662153));
#11841=CARTESIAN_POINT('Ctrl Pts',(16.1726398919203,118.293920461934,-35.1004804618895));
#11842=CARTESIAN_POINT('Ctrl Pts',(18.4055652335539,120.914492495622,-33.3636845708006));
#11843=CARTESIAN_POINT('Ctrl Pts',(19.7140335926606,122.06366179469,-32.2010375455974));
#11844=CARTESIAN_POINT('Ctrl Pts',(21.5995664992349,123.221455351176,-30.0976214728539));
#11845=CARTESIAN_POINT('Ctrl Pts',(22.2160215790544,123.516564269284,-29.3376278707406));
#11846=CARTESIAN_POINT('Ctrl Pts',(23.3708344330195,123.90590570748,-27.7463980926541));
#11847=CARTESIAN_POINT('Ctrl Pts',(23.9091058947705,124.,-26.9150654608326));
#11848=CARTESIAN_POINT('Ctrl Pts',(24.8713785355745,124.,-25.2483603562266));
#11849=CARTESIAN_POINT('Ctrl Pts',(25.3221979828513,123.90590570748,-24.3665372803074));
#11850=CARTESIAN_POINT('Ctrl Pts',(26.1228369669499,123.516564269284,-22.5708251231135));
#11851=CARTESIAN_POINT('Ctrl Pts',(26.4727831931839,123.221455351176,-21.6569625626412));
#11852=CARTESIAN_POINT('Ctrl Pts',(27.3516284936211,122.06366179469,-18.9723351295045));
#11853=CARTESIAN_POINT('Ctrl Pts',(27.7042761735281,120.914492495622,-17.2578447778684));
#11854=CARTESIAN_POINT('Ctrl Pts',(28.0919228655827,118.293920461934,-14.4556767617152));
#11855=CARTESIAN_POINT('Ctrl Pts',(28.1530911675774,116.634335598937,-13.1680461599312));
#11856=CARTESIAN_POINT('Ctrl Pts',(28.1664515850802,113.875241073532,-11.8413428056788));
#11857=CARTESIAN_POINT('Ctrl Pts',(28.1598618611454,112.910670985819,-11.4970448203705));
#11858=CARTESIAN_POINT('Ctrl Pts',(28.1479913014721,110.955993689506,-11.0401198405521));
#11859=CARTESIAN_POINT('Ctrl Pts',(28.1430112947403,109.965797205724,-10.9278670711359));
#11860=CARTESIAN_POINT('Ctrl Pts',(28.1430112947403,109.,-10.9278670711359));
#11861=CARTESIAN_POINT('Ctrl Pts',(28.1430112947403,109.,-10.9278670711359));
#11862=CARTESIAN_POINT('Ctrl Pts',(28.1430112947403,108.034202794276,-10.9278670711359));
#11863=CARTESIAN_POINT('Ctrl Pts',(28.1479913014721,107.044006310494,-11.0401198405521));
#11864=CARTESIAN_POINT('Ctrl Pts',(28.1598618611454,105.089329014181,-11.4970448203705));
#11865=CARTESIAN_POINT('Ctrl Pts',(28.1664515850802,104.124758926468,-11.8413428056788));
#11866=CARTESIAN_POINT('Ctrl Pts',(28.1530911675774,101.365664401063,-13.1680461599312));
#11867=CARTESIAN_POINT('Ctrl Pts',(28.0919228655827,99.7060795380662,-14.4556767617152));
#11868=CARTESIAN_POINT('Ctrl Pts',(27.7042761735281,97.0855075043779,-17.2578447778684));
#11869=CARTESIAN_POINT('Ctrl Pts',(27.3516284936211,95.9363382053097,-18.9723351295045));
#11870=CARTESIAN_POINT('Ctrl Pts',(26.4727831931839,94.7785446488243,-21.6569625626412));
#11871=CARTESIAN_POINT('Ctrl Pts',(26.1228369669499,94.4834357307163,-22.5708251231135));
#11872=CARTESIAN_POINT('Ctrl Pts',(25.3221979828513,94.0940942925199,-24.3665372803074));
#11873=CARTESIAN_POINT('Ctrl Pts',(24.8713785355745,94.,-25.2483603562266));
#11874=CARTESIAN_POINT('Ctrl Pts',(23.9091058947705,94.,-26.9150654608326));
#11875=CARTESIAN_POINT('Ctrl Pts',(23.3708344330195,94.0940942925199,-27.7463980926541));
#11876=CARTESIAN_POINT('Ctrl Pts',(22.2160215790544,94.4834357307163,-29.3376278707406));
#11877=CARTESIAN_POINT('Ctrl Pts',(21.5995664992349,94.7785446488243,-30.0976214728539));
#11878=CARTESIAN_POINT('Ctrl Pts',(19.7140335926605,95.9363382053097,-32.2010375455974));
#11879=CARTESIAN_POINT('Ctrl Pts',(18.4055652335539,97.0855075043779,-33.3636845708006));
#11880=CARTESIAN_POINT('Ctrl Pts',(16.1726398919203,99.7060795380662,-35.1004804618895));
#11881=CARTESIAN_POINT('Ctrl Pts',(15.0881032310825,101.365664401063,-35.7972690662153));
#11882=CARTESIAN_POINT('Ctrl Pts',(13.9458246317653,104.124758926468,-36.4721912043041));
#11883=CARTESIAN_POINT('Ctrl Pts',(13.6443589680491,105.089329014181,-36.6386333286268));
#11884=CARTESIAN_POINT('Ctrl Pts',(13.242715048066,107.044006310494,-36.8568156123018));
#11885=CARTESIAN_POINT('Ctrl Pts',(13.1430112947406,108.034202794276,-36.9086291846692));
#11886=CARTESIAN_POINT('Ctrl Pts',(13.1430112947406,109.,-36.9086291846692));
#11887=CARTESIAN_POINT('Origin',(0.,126.,-11.9999999999999));
#11888=CARTESIAN_POINT('',(-2.83670152841496E-15,126.,-35.1634258170598));
#11889=CARTESIAN_POINT('Origin',(0.,126.,-11.9999999999999));
#11890=CARTESIAN_POINT('Origin',(0.,89.,-11.9999999999999));
#11891=CARTESIAN_POINT('',(-2.44929359829471E-15,89.,8.00000000000008));
#11892=CARTESIAN_POINT('Origin',(0.,89.,-11.9999999999999));
#11893=CARTESIAN_POINT('Origin',(0.,125.,-11.9999999999999));
#11894=CARTESIAN_POINT('',(-2.83670152841496E-15,125.,-35.1634258170598));
#11895=CARTESIAN_POINT('Origin',(0.,125.,-11.9999999999999));
#11896=CARTESIAN_POINT('',(-2.83670152841496E-15,125.,-35.1634258170598));
#11897=CARTESIAN_POINT('Origin',(0.,125.,-11.9999999999999));
#11898=CARTESIAN_POINT('Origin',(4.79810263127257E-15,109.,-191.42723747195));
#11899=CARTESIAN_POINT('',(-15.,109.,57.5));
#11900=CARTESIAN_POINT('Origin',(4.79810263127257E-15,109.,57.5));
#11901=CARTESIAN_POINT('',(-15.,109.,-191.42723747195));
#11902=CARTESIAN_POINT('Origin',(4.79810263127257E-15,109.,61.5));
#11903=CARTESIAN_POINT('',(17.,109.,61.5));
#11904=CARTESIAN_POINT('Origin',(4.79810263127257E-15,109.,61.5));
#11905=CARTESIAN_POINT('',(-8.58443001961159,97.9916127703239,61.5));
#11906=CARTESIAN_POINT('',(-8.58443001961159,97.9916127703239,61.5));
#11907=CARTESIAN_POINT('',(-9.35047446273056,98.6344003800105,61.5));
#11908=CARTESIAN_POINT('',(-8.58443001961159,97.9916127703239,61.5));
#11909=CARTESIAN_POINT('',(-9.35047446273056,98.6344003800105,61.5));
#11910=CARTESIAN_POINT('',(-5.2413279857898,121.938528088831,61.5));
#11911=CARTESIAN_POINT('',(-5.2413279857898,121.938528088831,61.5));
#11912=CARTESIAN_POINT('',(-4.30163536500389,122.280548232157,61.5));
#11913=CARTESIAN_POINT('',(-5.2413279857898,121.938528088831,61.5));
#11914=CARTESIAN_POINT('',(-4.30163536500389,122.280548232157,61.5));
#11915=CARTESIAN_POINT('',(13.8257580054015,107.069859140845,61.5));
#11916=CARTESIAN_POINT('',(13.8257580054015,107.069859140845,61.5));
#11917=CARTESIAN_POINT('',(13.6521098277345,106.085051387833,61.5));
#11918=CARTESIAN_POINT('',(13.8257580054015,107.069859140845,61.5));
#11919=CARTESIAN_POINT('',(13.6521098277345,106.085051387833,61.5));
#11920=CARTESIAN_POINT('Origin',(4.79810263127257E-15,109.,61.5));
#11921=CARTESIAN_POINT('',(17.,109.,59.5));
#11922=CARTESIAN_POINT('',(-17.,109.,59.5));
#11923=CARTESIAN_POINT('Origin',(4.79810263127257E-15,109.,59.5));
#11924=CARTESIAN_POINT('Origin',(4.79810263127257E-15,109.,59.5));
#11925=CARTESIAN_POINT('',(17.,109.,61.5));
#11926=CARTESIAN_POINT('Origin',(4.79810263127257E-15,109.,-191.42723747195));
#11927=CARTESIAN_POINT('',(12.999999999998,109.,3.19868415357247));
#11928=CARTESIAN_POINT('',(3.63257893358771E-15,122.,8.00000000000008));
#11929=CARTESIAN_POINT('Ctrl Pts',(13.,109.,3.19868415357074));
#11930=CARTESIAN_POINT('Ctrl Pts',(13.,109.851995783248,3.19868415357074));
#11931=CARTESIAN_POINT('Ctrl Pts',(12.9150719143893,110.718692707522,3.27253856324928));
#11932=CARTESIAN_POINT('Ctrl Pts',(12.5720677115743,112.41995630624,3.55611229413735));
#11933=CARTESIAN_POINT('Ctrl Pts',(12.3141919444307,113.25470217185,3.76499824413062));
#11934=CARTESIAN_POINT('Ctrl Pts',(11.3107639081373,115.63581455956,4.51558245123477));
#11935=CARTESIAN_POINT('Ctrl Pts',(10.3239083354049,117.060867975445,5.17673327565937));
#11936=CARTESIAN_POINT('Ctrl Pts',(8.07178308824895,119.312993222601,6.34225725186619));
#11937=CARTESIAN_POINT('Ctrl Pts',(6.64417608295783,120.307169987275,6.93603058768733));
#11938=CARTESIAN_POINT('Ctrl Pts',(4.25116977785989,121.315715660585,7.56034611361149));
#11939=CARTESIAN_POINT('Ctrl Pts',(3.41196563272457,121.574314859725,7.72552166608632));
#11940=CARTESIAN_POINT('Ctrl Pts',(1.70829130581225,121.916526022509,7.94541188586552));
#11941=CARTESIAN_POINT('Ctrl Pts',(0.843777078670328,122.,8.00000000000008));
#11942=CARTESIAN_POINT('Ctrl Pts',(9.15933995315754E-15,122.,8.00000000000008));
#11943=CARTESIAN_POINT('',(2.43541035559477E-17,96.,8.00000000000008));
#11944=CARTESIAN_POINT('Ctrl Pts',(1.94289029309402E-15,96.,8.00000000000008));
#11945=CARTESIAN_POINT('Ctrl Pts',(0.84377707867032,96.,8.00000000000008));
#11946=CARTESIAN_POINT('Ctrl Pts',(1.70829130581224,96.0834739774908,7.94541188586552));
#11947=CARTESIAN_POINT('Ctrl Pts',(3.41196563272457,96.4256851402753,7.72552166608632));
#11948=CARTESIAN_POINT('Ctrl Pts',(4.25116977785989,96.6842843394153,7.56034611361149));
#11949=CARTESIAN_POINT('Ctrl Pts',(6.64417608295782,97.692830012725,6.93603058768733));
#11950=CARTESIAN_POINT('Ctrl Pts',(8.07178308824894,98.6870067773987,6.3422572518662));
#11951=CARTESIAN_POINT('Ctrl Pts',(10.3239083354049,100.939132024555,5.17673327565937));
#11952=CARTESIAN_POINT('Ctrl Pts',(11.3107639081373,102.36418544044,4.51558245123478));
#11953=CARTESIAN_POINT('Ctrl Pts',(12.3141919444307,104.74529782815,3.76499824413063));
#11954=CARTESIAN_POINT('Ctrl Pts',(12.5720677115743,105.58004369376,3.55611229413735));
#11955=CARTESIAN_POINT('Ctrl Pts',(12.9150719143893,107.281307292478,3.27253856324928));
#11956=CARTESIAN_POINT('Ctrl Pts',(13.,108.148004216753,3.19868415357074));
#11957=CARTESIAN_POINT('Ctrl Pts',(13.,109.,3.19868415357074));
#11958=CARTESIAN_POINT('',(-13.,109.,3.19868415357075));
#11959=CARTESIAN_POINT('Ctrl Pts',(-13.,109.,3.19868415357075));
#11960=CARTESIAN_POINT('Ctrl Pts',(-13.,108.148004216753,3.19868415357075));
#11961=CARTESIAN_POINT('Ctrl Pts',(-12.9150719143893,107.281307292478,3.27253856324928));
#11962=CARTESIAN_POINT('Ctrl Pts',(-12.5720677115743,105.58004369376,3.55611229413736));
#11963=CARTESIAN_POINT('Ctrl Pts',(-12.3141919444307,104.74529782815,3.76499824413063));
#11964=CARTESIAN_POINT('Ctrl Pts',(-11.3107639081373,102.36418544044,4.51558245123478));
#11965=CARTESIAN_POINT('Ctrl Pts',(-10.3239083354049,100.939132024555,5.17673327565937));
#11966=CARTESIAN_POINT('Ctrl Pts',(-8.07178308824894,98.6870067773987,6.3422572518662));
#11967=CARTESIAN_POINT('Ctrl Pts',(-6.64417608295782,97.692830012725,6.93603058768733));
#11968=CARTESIAN_POINT('Ctrl Pts',(-4.25116977785988,96.6842843394153,7.5603461136115));
#11969=CARTESIAN_POINT('Ctrl Pts',(-3.41196563272456,96.4256851402753,7.72552166608632));
#11970=CARTESIAN_POINT('Ctrl Pts',(-1.70829130581224,96.0834739774908,7.94541188586552));
#11971=CARTESIAN_POINT('Ctrl Pts',(-0.843777078670316,96.,8.00000000000008));
#11972=CARTESIAN_POINT('Ctrl Pts',(2.4980018054066E-15,96.,8.00000000000008));
#11973=CARTESIAN_POINT('',(-13.,109.,-191.42723747195));
#11974=CARTESIAN_POINT('Ctrl Pts',(8.60422844084496E-15,122.,8.00000000000008));
#11975=CARTESIAN_POINT('Ctrl Pts',(-0.843777078670309,122.,8.00000000000008));
#11976=CARTESIAN_POINT('Ctrl Pts',(-1.70829130581223,121.916526022509,7.94541188586552));
#11977=CARTESIAN_POINT('Ctrl Pts',(-3.41196563272456,121.574314859725,7.72552166608632));
#11978=CARTESIAN_POINT('Ctrl Pts',(-4.25116977785987,121.315715660585,7.5603461136115));
#11979=CARTESIAN_POINT('Ctrl Pts',(-6.64417608295781,120.307169987275,6.93603058768734));
#11980=CARTESIAN_POINT('Ctrl Pts',(-8.07178308824893,119.312993222601,6.3422572518662));
#11981=CARTESIAN_POINT('Ctrl Pts',(-10.3239083354049,117.060867975445,5.17673327565938));
#11982=CARTESIAN_POINT('Ctrl Pts',(-11.3107639081373,115.63581455956,4.51558245123479));
#11983=CARTESIAN_POINT('Ctrl Pts',(-12.3141919444307,113.25470217185,3.76499824413064));
#11984=CARTESIAN_POINT('Ctrl Pts',(-12.5720677115743,112.41995630624,3.55611229413736));
#11985=CARTESIAN_POINT('Ctrl Pts',(-12.9150719143893,110.718692707522,3.27253856324929));
#11986=CARTESIAN_POINT('Ctrl Pts',(-13.,109.851995783248,3.19868415357075));
#11987=CARTESIAN_POINT('Ctrl Pts',(-13.,109.,3.19868415357075));
#11988=CARTESIAN_POINT('Origin',(4.79810263127257E-15,109.,59.5));
#11989=CARTESIAN_POINT('',(-17.,109.,59.5));
#11990=CARTESIAN_POINT('Origin',(-54.6822367721436,109.,19.5708041202874));
#11991=CARTESIAN_POINT('',(67.6887655630186,109.,-33.7596189432327));
#11992=CARTESIAN_POINT('Origin',(60.1887655630187,109.,-46.7499999999993));
#11993=CARTESIAN_POINT('',(-47.1822367721437,109.,32.561185177054));
#11994=CARTESIAN_POINT('Origin',(54.6822367721438,109.,19.5708041202885));
#11995=CARTESIAN_POINT('',(-52.6887655630182,109.,-59.7403810567667));
#11996=CARTESIAN_POINT('Origin',(-60.1887655630183,109.,-46.7500000000002));
#11997=CARTESIAN_POINT('',(62.1822367721439,109.,6.58042306352195));
#11998=CARTESIAN_POINT('Origin',(-63.6528671781565,109.,-48.7499999999993));
#11999=CARTESIAN_POINT('',(-72.1528671781564,109.,-34.0275681356638));
#12000=CARTESIAN_POINT('Origin',(-63.6528671781565,109.,-48.7499999999993));
#12001=CARTESIAN_POINT('',(-61.5020494956546,122.280548232157,-52.4753255039102));
#12002=CARTESIAN_POINT('',(-61.5020494956546,122.280548232157,-52.4753255039102));
#12003=CARTESIAN_POINT('',(-70.5657461808571,107.069859140845,-36.7765423407455));
#12004=CARTESIAN_POINT('',(-70.5657461808571,107.069859140845,-36.7765423407455));
#12005=CARTESIAN_POINT('',(-70.4789220920237,106.085051387833,-36.9269260739259));
#12006=CARTESIAN_POINT('',(-70.5657461808571,107.069859140845,-36.7765423407455));
#12007=CARTESIAN_POINT('',(-70.4789220920237,106.085051387833,-36.9269260739259));
#12008=CARTESIAN_POINT('',(-59.3606521683508,97.9916127703239,-56.1843344739927));
#12009=CARTESIAN_POINT('',(-59.3606521683508,97.9916127703239,-56.1843344739927));
#12010=CARTESIAN_POINT('',(-58.9776299467913,98.6344003800105,-56.8477484221616));
#12011=CARTESIAN_POINT('',(-59.3606521683508,97.9916127703239,-56.1843344739927));
#12012=CARTESIAN_POINT('',(-58.9776299467913,98.6344003800105,-56.8477484221616));
#12013=CARTESIAN_POINT('',(-61.0322031852617,121.938528088831,-53.2891231852596));
#12014=CARTESIAN_POINT('',(-61.0322031852617,121.938528088831,-53.2891231852596));
#12015=CARTESIAN_POINT('',(-61.0322031852617,121.938528088831,-53.2891231852596));
#12016=CARTESIAN_POINT('Origin',(-63.6528671781565,109.,-48.7499999999993));
#12017=CARTESIAN_POINT('',(-70.4208163705874,109.,-33.0275681356637));
#12018=CARTESIAN_POINT('',(-53.4208163705878,109.,-62.4724318643349));
#12019=CARTESIAN_POINT('Origin',(-61.9208163705876,109.,-47.7499999999993));
#12020=CARTESIAN_POINT('Origin',(-61.9208163705876,109.,-47.7499999999993));
#12021=CARTESIAN_POINT('',(-72.1528671781564,109.,-34.0275681356638));
#12022=CARTESIAN_POINT('Origin',(63.652867178156,109.,-48.7500000000002));
#12023=CARTESIAN_POINT('',(55.152867178156,109.,-63.4724318643356));
#12024=CARTESIAN_POINT('Origin',(63.652867178156,109.,-48.7500000000002));
#12025=CARTESIAN_POINT('',(65.803684860658,122.280548232157,-45.0246744960893));
#12026=CARTESIAN_POINT('',(65.803684860658,122.280548232157,-45.0246744960893));
#12027=CARTESIAN_POINT('',(56.7399881754552,107.069859140845,-60.7234576592539));
#12028=CARTESIAN_POINT('',(56.7399881754552,107.069859140845,-60.7234576592539));
#12029=CARTESIAN_POINT('',(56.8268122642887,106.085051387833,-60.5730739260735));
#12030=CARTESIAN_POINT('',(56.7399881754552,107.069859140845,-60.7234576592539));
#12031=CARTESIAN_POINT('',(56.8268122642887,106.085051387833,-60.5730739260735));
#12032=CARTESIAN_POINT('',(67.9450821879618,97.991612770324,-41.3156655260068));
#12033=CARTESIAN_POINT('',(67.9450821879618,97.991612770324,-41.3156655260068));
#12034=CARTESIAN_POINT('',(68.3281044095213,98.6344003800105,-40.6522515778379));
#12035=CARTESIAN_POINT('',(67.9450821879618,97.991612770324,-41.3156655260068));
#12036=CARTESIAN_POINT('',(68.3281044095213,98.6344003800105,-40.6522515778379));
#12037=CARTESIAN_POINT('',(66.2735311710509,121.938528088831,-44.2108768147399));
#12038=CARTESIAN_POINT('',(66.2735311710509,121.938528088831,-44.2108768147399));
#12039=CARTESIAN_POINT('',(66.2735311710509,121.938528088831,-44.2108768147399));
#12040=CARTESIAN_POINT('Origin',(63.652867178156,109.,-48.7500000000002));
#12041=CARTESIAN_POINT('',(53.4208163705871,109.,-62.4724318643356));
#12042=CARTESIAN_POINT('',(70.4208163705872,109.,-33.0275681356648));
#12043=CARTESIAN_POINT('Origin',(61.9208163705871,109.,-47.7500000000002));
#12044=CARTESIAN_POINT('Origin',(61.9208163705871,109.,-47.7500000000002));
#12045=CARTESIAN_POINT('',(55.152867178156,109.,-63.4724318643356));
#12046=CARTESIAN_POINT('Origin',(84.3262415816127,109.,36.6857782768941));
#12047=CARTESIAN_POINT('',(-19.6624465810882,109.,-8.34101182758738));
#12048=CARTESIAN_POINT('',(-6.66244658108813,109.,-30.857672325983));
#12049=CARTESIAN_POINT('Ctrl Pts',(-19.6624465810882,109.,-8.34101182758764));
#12050=CARTESIAN_POINT('Ctrl Pts',(-19.6624465810882,109.851995783248,-8.34101182758764));
#12051=CARTESIAN_POINT('Ctrl Pts',(-19.683942333246,110.718692707522,-8.45148891206053));
#12052=CARTESIAN_POINT('Ctrl Pts',(-19.7580222866335,112.41995630624,-8.89032613074718));
#12053=CARTESIAN_POINT('Ctrl Pts',(-19.8099849422495,113.25470217185,-9.21809607111061));
#12054=CARTESIAN_POINT('Ctrl Pts',(-19.9582959151344,115.63581455956,-10.4623823449623));
#12055=CARTESIAN_POINT('Ctrl Pts',(-20.0374415384529,117.060867975445,-11.6475997530271));
#12056=CARTESIAN_POINT('Ctrl Pts',(-19.9207522869899,119.312993222601,-14.1807594176719));
#12057=CARTESIAN_POINT('Ctrl Pts',(-19.7211715772552,120.307169987275,-15.7139900187852));
#12058=CARTESIAN_POINT('Ctrl Pts',(-19.0653415301336,121.315715660585,-18.0985520333784));
#12059=CARTESIAN_POINT('Ctrl Pts',(-18.7887856820933,121.574314859725,-18.9079119182642));
#12060=CARTESIAN_POINT('Ctrl Pts',(-18.1273790350096,121.916526022509,-20.4932822750352));
#12061=CARTESIAN_POINT('Ctrl Pts',(-17.7423966150239,122.,-21.2692676147405));
#12062=CARTESIAN_POINT('Ctrl Pts',(-16.8986195363536,122.,-22.7307323852595));
#12063=CARTESIAN_POINT('Ctrl Pts',(-16.4190877291974,121.916526022509,-23.4521296108302));
#12064=CARTESIAN_POINT('Ctrl Pts',(-15.3768200493687,121.574314859725,-24.817609747822));
#12065=CARTESIAN_POINT('Ctrl Pts',(-14.8141717522737,121.315715660585,-25.461794080233));
#12066=CARTESIAN_POINT('Ctrl Pts',(-13.0769954942974,120.307169987275,-27.2220405689021));
#12067=CARTESIAN_POINT('Ctrl Pts',(-11.8489691987409,119.312993222601,-28.1614978341942));
#12068=CARTESIAN_POINT('Ctrl Pts',(-9.71353320304791,117.060867975445,-29.5291335226322));
#12069=CARTESIAN_POINT('Ctrl Pts',(-8.647532006997,115.63581455956,-30.0532001062724));
#12070=CARTESIAN_POINT('Ctrl Pts',(-7.49579299781871,113.25470217185,-30.5469021730199));
#12071=CARTESIAN_POINT('Ctrl Pts',(-7.18595457505908,112.41995630624,-30.66578616339));
#12072=CARTESIAN_POINT('Ctrl Pts',(-6.76887041885657,110.718692707522,-30.8210496511886));
#12073=CARTESIAN_POINT('Ctrl Pts',(-6.6624465810881,109.851995783248,-30.857672325983));
#12074=CARTESIAN_POINT('Ctrl Pts',(-6.6624465810881,109.,-30.857672325983));
#12075=CARTESIAN_POINT('Ctrl Pts',(-6.6624465810881,109.,-30.857672325983));
#12076=CARTESIAN_POINT('Ctrl Pts',(-6.6624465810881,108.148004216753,-30.857672325983));
#12077=CARTESIAN_POINT('Ctrl Pts',(-6.76887041885657,107.281307292478,-30.8210496511886));
#12078=CARTESIAN_POINT('Ctrl Pts',(-7.18595457505907,105.58004369376,-30.66578616339));
#12079=CARTESIAN_POINT('Ctrl Pts',(-7.4957929978187,104.74529782815,-30.5469021730199));
#12080=CARTESIAN_POINT('Ctrl Pts',(-8.64753200699699,102.36418544044,-30.0532001062724));
#12081=CARTESIAN_POINT('Ctrl Pts',(-9.7135332030479,100.939132024555,-29.5291335226322));
#12082=CARTESIAN_POINT('Ctrl Pts',(-11.8489691987408,98.6870067773987,-28.1614978341942));
#12083=CARTESIAN_POINT('Ctrl Pts',(-13.0769954942973,97.692830012725,-27.2220405689021));
#12084=CARTESIAN_POINT('Ctrl Pts',(-14.8141717522737,96.6842843394153,-25.461794080233));
#12085=CARTESIAN_POINT('Ctrl Pts',(-15.3768200493687,96.4256851402753,-24.817609747822));
#12086=CARTESIAN_POINT('Ctrl Pts',(-16.4190877291974,96.0834739774908,-23.4521296108302));
#12087=CARTESIAN_POINT('Ctrl Pts',(-16.8986195363536,96.,-22.7307323852595));
#12088=CARTESIAN_POINT('Ctrl Pts',(-17.7423966150239,96.,-21.2692676147405));
#12089=CARTESIAN_POINT('Ctrl Pts',(-18.1273790350096,96.0834739774909,-20.4932822750352));
#12090=CARTESIAN_POINT('Ctrl Pts',(-18.7887856820933,96.4256851402753,-18.9079119182642));
#12091=CARTESIAN_POINT('Ctrl Pts',(-19.0653415301336,96.6842843394153,-18.0985520333784));
#12092=CARTESIAN_POINT('Ctrl Pts',(-19.7211715772552,97.692830012725,-15.7139900187852));
#12093=CARTESIAN_POINT('Ctrl Pts',(-19.9207522869899,98.6870067773987,-14.1807594176719));
#12094=CARTESIAN_POINT('Ctrl Pts',(-20.0374415384529,100.939132024555,-11.6475997530271));
#12095=CARTESIAN_POINT('Ctrl Pts',(-19.9582959151344,102.36418544044,-10.4623823449623));
#12096=CARTESIAN_POINT('Ctrl Pts',(-19.8099849422495,104.74529782815,-9.21809607111062));
#12097=CARTESIAN_POINT('Ctrl Pts',(-19.7580222866335,105.58004369376,-8.8903261307472));
#12098=CARTESIAN_POINT('Ctrl Pts',(-19.683942333246,107.281307292478,-8.45148891206054));
#12099=CARTESIAN_POINT('Ctrl Pts',(-19.6624465810882,108.148004216753,-8.34101182758764));
#12100=CARTESIAN_POINT('Ctrl Pts',(-19.6624465810882,109.,-8.34101182758764));
#12101=CARTESIAN_POINT('',(90.8262415816127,109.,25.4274480276964));
#12102=CARTESIAN_POINT('Origin',(-84.3262415816127,109.,36.6857782768926));
#12103=CARTESIAN_POINT('',(6.66244658108983,109.,-30.8576723259824));
#12104=CARTESIAN_POINT('',(19.6624465810882,109.,-8.34101182758737));
#12105=CARTESIAN_POINT('Ctrl Pts',(6.66244658108836,109.,-30.8576723259829));
#12106=CARTESIAN_POINT('Ctrl Pts',(6.66244658108836,109.851995783247,-30.8576723259829));
#12107=CARTESIAN_POINT('Ctrl Pts',(6.76887041885683,110.718692707522,-30.8210496511885));
#12108=CARTESIAN_POINT('Ctrl Pts',(7.18595457505932,112.41995630624,-30.6657861633899));
#12109=CARTESIAN_POINT('Ctrl Pts',(7.49579299781897,113.25470217185,-30.5469021730198));
#12110=CARTESIAN_POINT('Ctrl Pts',(8.64753200699724,115.63581455956,-30.0532001062722));
#12111=CARTESIAN_POINT('Ctrl Pts',(9.71353320304815,117.060867975445,-29.5291335226321));
#12112=CARTESIAN_POINT('Ctrl Pts',(11.8489691987411,119.312993222601,-28.1614978341941));
#12113=CARTESIAN_POINT('Ctrl Pts',(13.0769954942976,120.307169987275,-27.2220405689019));
#12114=CARTESIAN_POINT('Ctrl Pts',(14.8141717522739,121.315715660585,-25.4617940802328));
#12115=CARTESIAN_POINT('Ctrl Pts',(15.3768200493689,121.574314859725,-24.8176097478218));
#12116=CARTESIAN_POINT('Ctrl Pts',(16.4190877291975,121.916526022509,-23.45212961083));
#12117=CARTESIAN_POINT('Ctrl Pts',(16.8986195363537,122.,-22.7307323852593));
#12118=CARTESIAN_POINT('Ctrl Pts',(17.742396615024,122.,-21.2692676147402));
#12119=CARTESIAN_POINT('Ctrl Pts',(18.1273790350098,121.916526022509,-20.493282275035));
#12120=CARTESIAN_POINT('Ctrl Pts',(18.7887856820934,121.574314859725,-18.9079119182639));
#12121=CARTESIAN_POINT('Ctrl Pts',(19.0653415301337,121.315715660585,-18.0985520333781));
#12122=CARTESIAN_POINT('Ctrl Pts',(19.7211715772553,120.307169987275,-15.7139900187849));
#12123=CARTESIAN_POINT('Ctrl Pts',(19.9207522869899,119.312993222601,-14.1807594176716));
#12124=CARTESIAN_POINT('Ctrl Pts',(20.0374415384529,117.060867975445,-11.6475997530268));
#12125=CARTESIAN_POINT('Ctrl Pts',(19.9582959151344,115.63581455956,-10.462382344962));
#12126=CARTESIAN_POINT('Ctrl Pts',(19.8099849422494,113.25470217185,-9.21809607111035));
#12127=CARTESIAN_POINT('Ctrl Pts',(19.7580222866334,112.41995630624,-8.89032613074693));
#12128=CARTESIAN_POINT('Ctrl Pts',(19.6839423332459,110.718692707522,-8.45148891206027));
#12129=CARTESIAN_POINT('Ctrl Pts',(19.6624465810881,109.851995783248,-8.34101182758737));
#12130=CARTESIAN_POINT('Ctrl Pts',(19.6624465810881,109.,-8.34101182758737));
#12131=CARTESIAN_POINT('Ctrl Pts',(19.6624465810881,109.,-8.34101182758737));
#12132=CARTESIAN_POINT('Ctrl Pts',(19.6624465810881,108.148004216753,-8.34101182758737));
#12133=CARTESIAN_POINT('Ctrl Pts',(19.6839423332459,107.281307292478,-8.45148891206027));
#12134=CARTESIAN_POINT('Ctrl Pts',(19.7580222866334,105.58004369376,-8.89032613074692));
#12135=CARTESIAN_POINT('Ctrl Pts',(19.8099849422494,104.74529782815,-9.21809607111035));
#12136=CARTESIAN_POINT('Ctrl Pts',(19.9582959151344,102.36418544044,-10.462382344962));
#12137=CARTESIAN_POINT('Ctrl Pts',(20.0374415384529,100.939132024555,-11.6475997530268));
#12138=CARTESIAN_POINT('Ctrl Pts',(19.9207522869899,98.6870067773987,-14.1807594176716));
#12139=CARTESIAN_POINT('Ctrl Pts',(19.7211715772553,97.692830012725,-15.7139900187849));
#12140=CARTESIAN_POINT('Ctrl Pts',(19.0653415301337,96.6842843394153,-18.0985520333781));
#12141=CARTESIAN_POINT('Ctrl Pts',(18.7887856820934,96.4256851402753,-18.9079119182639));
#12142=CARTESIAN_POINT('Ctrl Pts',(18.1273790350098,96.0834739774908,-20.493282275035));
#12143=CARTESIAN_POINT('Ctrl Pts',(17.742396615024,96.,-21.2692676147402));
#12144=CARTESIAN_POINT('Ctrl Pts',(16.8986195363537,96.,-22.7307323852593));
#12145=CARTESIAN_POINT('Ctrl Pts',(16.4190877291975,96.0834739774908,-23.45212961083));
#12146=CARTESIAN_POINT('Ctrl Pts',(15.3768200493689,96.4256851402753,-24.8176097478218));
#12147=CARTESIAN_POINT('Ctrl Pts',(14.8141717522739,96.6842843394153,-25.4617940802328));
#12148=CARTESIAN_POINT('Ctrl Pts',(13.0769954942976,97.692830012725,-27.2220405689019));
#12149=CARTESIAN_POINT('Ctrl Pts',(11.8489691987411,98.6870067773987,-28.1614978341941));
#12150=CARTESIAN_POINT('Ctrl Pts',(9.71353320304814,100.939132024555,-29.5291335226321));
#12151=CARTESIAN_POINT('Ctrl Pts',(8.64753200699724,102.36418544044,-30.0532001062722));
#12152=CARTESIAN_POINT('Ctrl Pts',(7.49579299781896,104.74529782815,-30.5469021730198));
#12153=CARTESIAN_POINT('Ctrl Pts',(7.18595457505932,105.58004369376,-30.6657861633899));
#12154=CARTESIAN_POINT('Ctrl Pts',(6.76887041885682,107.281307292478,-30.8210496511885));
#12155=CARTESIAN_POINT('Ctrl Pts',(6.66244658108837,108.148004216753,-30.8576723259829));
#12156=CARTESIAN_POINT('Ctrl Pts',(6.66244658108837,109.,-30.8576723259829));
#12157=CARTESIAN_POINT('',(-77.8262415816128,109.,47.9441085260903));
#12158=CARTESIAN_POINT('Origin',(61.9208163705871,109.,-47.7500000000002));
#12159=CARTESIAN_POINT('',(70.4208163705872,109.,-33.0275681356648));
#12160=CARTESIAN_POINT('Origin',(-61.9208163705876,109.,-47.7499999999993));
#12161=CARTESIAN_POINT('',(-53.4208163705878,109.,-62.4724318643349));
#12162=CARTESIAN_POINT('Origin',(0.,123.,-11.9999999999999));
#12163=CARTESIAN_POINT('',(0.,123.,8.00000000000008));
#12164=CARTESIAN_POINT('Origin',(0.,123.,-11.9999999999999));
#12165=CARTESIAN_POINT('Origin',(0.,181.568542494924,-11.9999999999999));
#12166=CARTESIAN_POINT('',(-2.44929359829471E-15,181.568542494924,8.00000000000008));
#12167=CARTESIAN_POINT('',(-2.44929359829471E-15,181.568542494924,8.00000000000008));
#12168=CARTESIAN_POINT('Origin',(-4.30163536500389,122.280548232157,61.5));
#12169=CARTESIAN_POINT('',(-4.30163536500389,122.280548232157,61.5));
#12170=CARTESIAN_POINT('Origin',(-5.2413279857898,121.938528088831,61.5));
#12171=CARTESIAN_POINT('',(-5.2413279857898,121.938528088831,65.5));
#12172=CARTESIAN_POINT('Origin',(-39.8034064033113,109.35896031048,0.));
#12173=CARTESIAN_POINT('Origin',(13.6521098277345,106.085051387833,61.5));
#12174=CARTESIAN_POINT('',(13.6521098277345,106.085051387833,61.5));
#12175=CARTESIAN_POINT('Origin',(13.8257580054015,107.069859140845,61.5));
#12176=CARTESIAN_POINT('',(13.8257580054015,107.069859140845,65.5));
#12177=CARTESIAN_POINT('Origin',(20.2125719494813,143.291280947184,0.));
#12178=CARTESIAN_POINT('Origin',(-9.35047446273056,98.6344003800105,61.5));
#12179=CARTESIAN_POINT('',(-9.35047446273056,98.6344003800105,61.5));
#12180=CARTESIAN_POINT('Origin',(-8.58443001961159,97.9916127703239,61.5));
#12181=CARTESIAN_POINT('',(-8.58443001961159,97.9916127703239,65.5));
#12182=CARTESIAN_POINT('Origin',(19.5908344538299,74.3497587423363,0.));
#12183=CARTESIAN_POINT('Origin',(56.8268122642887,106.085051387833,-60.5730739260735));
#12184=CARTESIAN_POINT('',(56.8268122642887,106.085051387833,-60.5730739260735));
#12185=CARTESIAN_POINT('Origin',(56.7399881754552,107.069859140845,-60.7234576592539));
#12186=CARTESIAN_POINT('',(60.204089790593,107.069859140845,-62.7234576592539));
#12187=CARTESIAN_POINT('Origin',(0.286018870672457,143.291280947184,-35.5046007840714));
#12188=CARTESIAN_POINT('Origin',(68.3281044095213,98.6344003800105,-40.6522515778379));
#12189=CARTESIAN_POINT('',(68.3281044095213,98.6344003800105,-40.6522515778379));
#12190=CARTESIAN_POINT('Origin',(67.9450821879618,97.991612770324,-41.3156655260068));
#12191=CARTESIAN_POINT('',(71.4091838030996,97.991612770324,-43.3156655260069));
#12192=CARTESIAN_POINT('Origin',(0.596887618498113,74.3497587423363,-34.9661603183521));
#12193=CARTESIAN_POINT('Origin',(65.803684860658,122.280548232157,-45.0246744960893));
#12194=CARTESIAN_POINT('',(65.803684860658,122.280548232157,-45.0246744960893));
#12195=CARTESIAN_POINT('Origin',(66.2735311710509,121.938528088831,-44.2108768147399));
#12196=CARTESIAN_POINT('',(69.7376327861887,121.938528088831,-46.2108768147399));
#12197=CARTESIAN_POINT('Origin',(30.294008047069,109.35896031048,16.4707611024238));
#12198=CARTESIAN_POINT('Origin',(-70.4789220920237,106.085051387833,-36.9269260739259));
#12199=CARTESIAN_POINT('',(-70.4789220920237,106.085051387833,-36.9269260739259));
#12200=CARTESIAN_POINT('Origin',(-70.5657461808571,107.069859140845,-36.7765423407455));
#12201=CARTESIAN_POINT('',(-74.0298477959949,107.069859140845,-38.7765423407454));
#12202=CARTESIAN_POINT('Origin',(-20.4985908201537,143.291280947184,-0.495399215928158));
#12203=CARTESIAN_POINT('Origin',(-58.9776299467913,98.6344003800105,-56.8477484221616));
#12204=CARTESIAN_POINT('',(-58.9776299467913,98.6344003800105,-56.8477484221616));
#12205=CARTESIAN_POINT('Origin',(-59.3606521683508,97.9916127703239,-56.1843344739927));
#12206=CARTESIAN_POINT('',(-62.8247537834886,97.9916127703239,-58.1843344739927));
#12207=CARTESIAN_POINT('Origin',(-20.1877220723281,74.3497587423363,-1.03383968164755));
#12208=CARTESIAN_POINT('Origin',(-61.5020494956546,122.280548232157,-52.4753255039102));
#12209=CARTESIAN_POINT('',(-61.5020494956546,122.280548232157,-52.4753255039102));
#12210=CARTESIAN_POINT('Origin',(-61.0322031852617,121.938528088831,-53.2891231852596));
#12211=CARTESIAN_POINT('',(-64.4963048003994,121.938528088831,-55.2891231852596));
#12212=CARTESIAN_POINT('Origin',(9.5093983562421,109.35896031048,-52.4707611024238));
#14105=UNCERTAINTY_MEASURE_WITH_UNIT(LENGTH_MEASURE(0.01),#14126,
'DISTANCE_ACCURACY_VALUE',
'Maximum model space distance between geometric entities at asserted c
onnectivities');
#14112=UNCERTAINTY_MEASURE_WITH_UNIT(LENGTH_MEASURE(0.01),#14126,
'DISTANCE_ACCURACY_VALUE',
'Maximum model space distance between geometric entities at asserted c
onnectivities');
#14118=(
GEOMETRIC_REPRESENTATION_CONTEXT(3)
GLOBAL_UNCERTAINTY_ASSIGNED_CONTEXT((#14105))
GLOBAL_UNIT_ASSIGNED_CONTEXT((#14126,#14128,#14129))
REPRESENTATION_CONTEXT('','3D')
);
#14125=(
GEOMETRIC_REPRESENTATION_CONTEXT(3)
GLOBAL_UNCERTAINTY_ASSIGNED_CONTEXT((#14112))
GLOBAL_UNIT_ASSIGNED_CONTEXT((#14126,#14128,#14129))
REPRESENTATION_CONTEXT('','3D')
);
#14126=(
LENGTH_UNIT()
NAMED_UNIT(*)
SI_UNIT(.MILLI.,.METRE.)
);
#14128=(
NAMED_UNIT(*)
PLANE_ANGLE_UNIT()
SI_UNIT($,.RADIAN.)
);
#14129=(
NAMED_UNIT(*)
SI_UNIT($,.STERADIAN.)
SOLID_ANGLE_UNIT()
);
#14135=SHAPE_DEFINITION_REPRESENTATION(#14147,#14204);
#14147=PRODUCT_DEFINITION_SHAPE('',$,#14217);
#14204=SHAPE_REPRESENTATION('',(#6478),#14118);
#14211=PRODUCT_DEFINITION_CONTEXT('part definition',#14249,'design');
#14217=PRODUCT_DEFINITION('Top','Top',#14229,#14211);
#14229=PRODUCT_DEFINITION_FORMATION('',$,#14256);
#14249=APPLICATION_CONTEXT(
'Core Data for Automotive Mechanical Design Process');
#14250=PRODUCT_CONTEXT('part definition',#14249,'mechanical');
#14256=PRODUCT('Top','Top',$,(#14250));
#14263=PRESENTATION_STYLE_ASSIGNMENT((#14265));
#14264=PRESENTATION_STYLE_ASSIGNMENT((#14266));
#14265=SURFACE_STYLE_USAGE(.BOTH.,#14267);
#14266=SURFACE_STYLE_USAGE(.BOTH.,#14268);
#14267=SURFACE_SIDE_STYLE('',(#14269));
#14268=SURFACE_SIDE_STYLE('',(#14270));
#14269=SURFACE_STYLE_FILL_AREA(#14271);
#14270=SURFACE_STYLE_FILL_AREA(#14272);
#14271=FILL_AREA_STYLE('Steel - Satin',(#14273));
#14272=FILL_AREA_STYLE('Opaque(255,255,255)',(#14274));
#14273=FILL_AREA_STYLE_COLOUR('Steel - Satin',#14275);
#14274=FILL_AREA_STYLE_COLOUR('Opaque(255,255,255)',#14276);
#14275=COLOUR_RGB('Steel - Satin',0.627450980392157,0.627450980392157,0.627450980392157);
#14276=COLOUR_RGB('Opaque(255,255,255)',1.,1.,1.);
ENDSEC;
END-ISO-10303-21;
